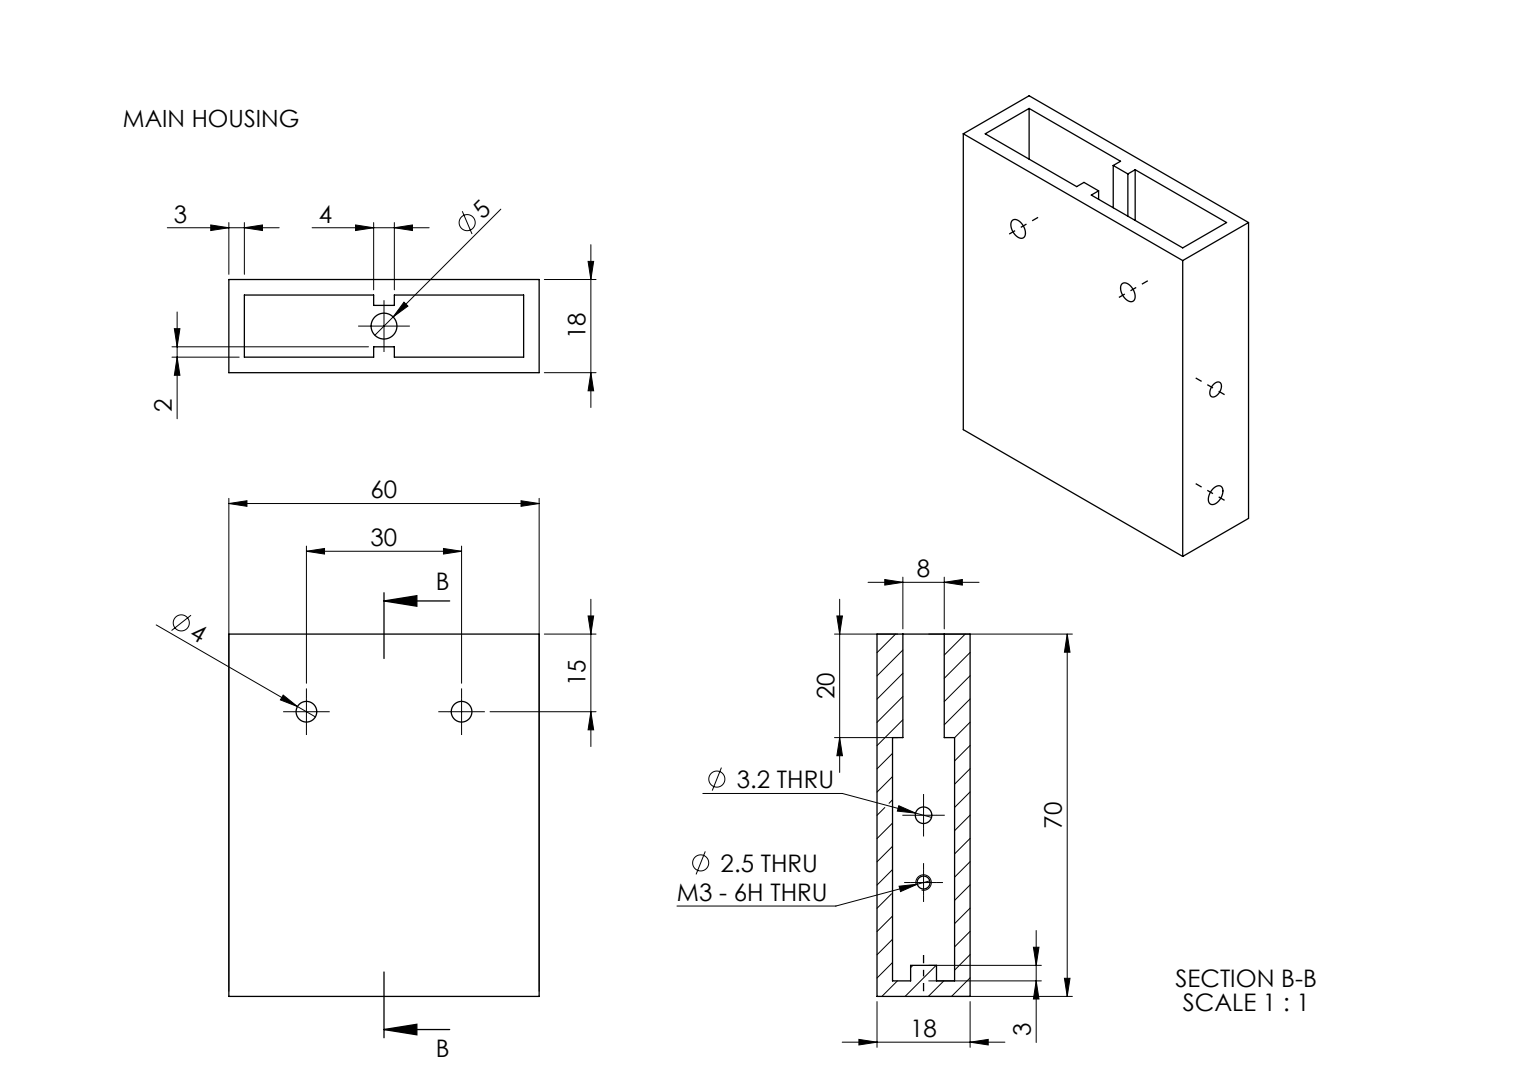
ISO-10303-21;
HEADER;
FILE_DESCRIPTION (('STEP AP214'),
    '1' );
FILE_NAME ('main housing.step',
    '2026-10-03T18:28:46',
    ( '' ),
    ( '' ),
    'SwSTEP 2.0',
    'SolidWorks 2026',
    '' );
FILE_SCHEMA (( 'AUTOMOTIVE_DESIGN' ));
ENDSEC;

DATA;
#38=CARTESIAN_POINT ( 'NONE',  ( 7.054542135639013677E-15, -28.99999999999999289, 0.000000000000000000 ) ) ;
#48=VERTEX_POINT ( 'NONE', #8977 ) ;
#68=DIRECTION ( 'NONE',  ( 0.000000000000000000, -0.000000000000000000, 1.000000000000000000 ) ) ;
#80=PRODUCT_DEFINITION_CONTEXT ( 'detailed design', #6135, 'design' ) ;
#82=PLANE ( 'NONE',  #8867 ) ;
#92=ORIENTED_EDGE ( 'NONE', *, *, #6887, .T. ) ;
#105=ORIENTED_EDGE ( 'NONE', *, *, #5645, .T. ) ;
#118=VERTEX_POINT ( 'NONE', #6579 ) ;
#125=CARTESIAN_POINT ( 'NONE',  ( 30.00000000000001066, -34.99999999999999289, -9.000000000000000000 ) ) ;
#137=DIRECTION ( 'NONE',  ( 5.204170427930421283E-15, 6.018531076210112041E-31, 1.000000000000000000 ) ) ;
#159=CARTESIAN_POINT ( 'NONE',  ( 1.999999999999987121, 15.00000000000000355, 4.000000000000008882 ) ) ;
#183=AXIS2_PLACEMENT_3D ( 'NONE', #2466, #1616, #8926 ) ;
#189=DIRECTION ( 'NONE',  ( 1.000000000000000000, 1.156482317317871478E-16, 5.637851296924623057E-15 ) ) ;
#199=VECTOR ( 'NONE', #189, 1000.000000000000000 ) ;
#205=DIRECTION ( 'NONE',  ( 0.000000000000000000, 0.000000000000000000, 1.000000000000000000 ) ) ;
#207=ORIENTED_EDGE ( 'NONE', *, *, #5389, .F. ) ;
#221=DIRECTION ( 'NONE',  ( -0.000000000000000000, -0.000000000000000000, 1.000000000000000000 ) ) ;
#225=CYLINDRICAL_SURFACE ( 'NONE', #1715, 2.500000000000000000 ) ;
#233=EDGE_CURVE ( 'NONE', #10188, #6283, #1978, .T. ) ;
#236=DIRECTION ( 'NONE',  ( -0.000000000000000000, -0.000000000000000000, 1.000000000000000000 ) ) ;
#269=ORIENTED_EDGE ( 'NONE', *, *, #2906, .F. ) ;
#278=PLANE ( 'NONE',  #8859 ) ;
#292=VERTEX_POINT ( 'NONE', #4247 ) ;
#294=DIRECTION ( 'NONE',  ( 0.000000000000000000, 0.000000000000000000, -1.000000000000000000 ) ) ;
#302=ORIENTED_EDGE ( 'NONE', *, *, #6506, .F. ) ;
#317=VERTEX_POINT ( 'NONE', #6837 ) ;
#322=ORIENTED_EDGE ( 'NONE', *, *, #3486, .F. ) ;
#331=DIRECTION ( 'NONE',  ( -1.000000000000000000, -4.625929269271485914E-16, 0.000000000000000000 ) ) ;
#341=VECTOR ( 'NONE', #1990, 1000.000000000000000 ) ;
#353=EDGE_CURVE ( 'NONE', #8450, #9806, #2322, .T. ) ;
#373=DIRECTION ( 'NONE',  ( 1.000000000000000000, -0.000000000000000000, -0.000000000000000000 ) ) ;
#386=CARTESIAN_POINT ( 'NONE',  ( 15.00000000000000000, 19.99999999999999645, -9.000000000000000000 ) ) ;
#397=AXIS2_PLACEMENT_3D ( 'NONE', #6365, #7050, #5039 ) ;
#398=EDGE_CURVE ( 'NONE', #7355, #525, #6229, .T. ) ;
#407=LINE ( 'NONE', #6055, #6780 ) ;
#409=VERTEX_POINT ( 'NONE', #6198 ) ;
#426=ORIENTED_EDGE ( 'NONE', *, *, #10066, .T. ) ;
#437=FACE_OUTER_BOUND ( 'NONE', #3682, .T. ) ;
#447=EDGE_CURVE ( 'NONE', #6622, #1459, #1384, .T. ) ;
#459=ORIENTED_EDGE ( 'NONE', *, *, #8953, .F. ) ;
#465=UNCERTAINTY_MEASURE_WITH_UNIT (LENGTH_MEASURE( 1.000000000000000082E-05 ), #9812, 'distance_accuracy_value', 'NONE');
#471=FACE_OUTER_BOUND ( 'NONE', #5653, .T. ) ;
#492=AXIS2_PLACEMENT_3D ( 'NONE', #2926, #2979, #637 ) ;
#512=ORIENTED_EDGE ( 'NONE', *, *, #4233, .T. ) ;
#516=AXIS2_PLACEMENT_3D ( 'NONE', #386, #236, #2717 ) ;
#522=VECTOR ( 'NONE', #7006, 1000.000000000000000 ) ;
#523=FACE_OUTER_BOUND ( 'NONE', #2494, .T. ) ;
#525=VERTEX_POINT ( 'NONE', #8496 ) ;
#530=ADVANCED_FACE ( 'NONE', ( #437 ), #3663, .F. ) ;
#533=SURFACE_SIDE_STYLE ('',( #7795 ) ) ;
#536=DIRECTION ( 'NONE',  ( 1.000000000000000000, 0.000000000000000000, 0.000000000000000000 ) ) ;
#541=EDGE_CURVE ( 'NONE', #3837, #9529, #1280, .T. ) ;
#556=ORIENTED_EDGE ( 'NONE', *, *, #8304, .F. ) ;
#565=EDGE_LOOP ( 'NONE', ( #3549, #2681, #8103, #9350 ) ) ;
#570=LINE ( 'NONE', #3276, #6753 ) ;
#576=CIRCLE ( 'NONE', #8201, 2.000000000000001776 ) ;
#585=CARTESIAN_POINT ( 'NONE',  ( 30.00000000000001066, -31.99999999999998579, 9.000000000000000000 ) ) ;
#597=LINE ( 'NONE', #648, #8239 ) ;
#617=DIRECTION ( 'NONE',  ( -0.000000000000000000, -0.000000000000000000, 1.000000000000000000 ) ) ;
#622=ORIENTED_EDGE ( 'NONE', *, *, #4233, .F. ) ;
#635=DIRECTION ( 'NONE',  ( -0.000000000000000000, -0.000000000000000000, 1.000000000000000000 ) ) ;
#636=FACE_BOUND ( 'NONE', #3921, .T. ) ;
#637=DIRECTION ( 'NONE',  ( 0.000000000000000000, 0.000000000000000000, 1.000000000000000000 ) ) ;
#648=CARTESIAN_POINT ( 'NONE',  ( 1.999999999999986233, 15.00000000000000355, -4.000000000000009770 ) ) ;
#659=ORIENTED_EDGE ( 'NONE', *, *, #7728, .T. ) ;
#662=ORIENTED_EDGE ( 'NONE', *, *, #2847, .T. ) ;
#668=AXIS2_PLACEMENT_3D ( 'NONE', #5379, #617, #3899 ) ;
#676=LINE ( 'NONE', #2269, #8398 ) ;
#681=DIRECTION ( 'NONE',  ( -1.156482317317871478E-16, 1.000000000000000000, 0.000000000000000000 ) ) ;
#688=SURFACE_STYLE_USAGE ( .BOTH. , #533 ) ;
#692=CARTESIAN_POINT ( 'NONE',  ( -2.000000000000015099, 35.00000000000000000, 3.999999999999986233 ) ) ;
#696=DIRECTION ( 'NONE',  ( -1.000000000000000000, -2.312964634635742957E-16, 0.000000000000000000 ) ) ;
#701=VECTOR ( 'NONE', #1350, 1000.000000000000000 ) ;
#713=DIRECTION ( 'NONE',  ( 1.156482317317871478E-16, -1.000000000000000000, 0.000000000000000000 ) ) ;
#714=CARTESIAN_POINT ( 'NONE',  ( -13.00000000000000000, 19.99999999999999645, -9.000000000000000000 ) ) ;
#724=ORIENTED_EDGE ( 'NONE', *, *, #8186, .F. ) ;
#730=AXIS2_PLACEMENT_3D ( 'NONE', #6023, #9492, #6879 ) ;
#746=FACE_OUTER_BOUND ( 'NONE', #9469, .T. ) ;
#761=DIRECTION ( 'NONE',  ( 4.625929269271485914E-16, -1.000000000000000000, 0.000000000000000000 ) ) ;
#762=CARTESIAN_POINT ( 'NONE',  ( 30.00000000000001066, 35.00000000000001421, 5.999999999999999112 ) ) ;
#772=ORIENTED_EDGE ( 'NONE', *, *, #3509, .F. ) ;
#778=CARTESIAN_POINT ( 'NONE',  ( -29.99999999999998934, -35.00000000000000000, 9.000000000000000000 ) ) ;
#781=VECTOR ( 'NONE', #5041, 1000.000000000000000 ) ;
#805=EDGE_LOOP ( 'NONE', ( #3050, #7525, #1781, #3634 ) ) ;
#834=LINE ( 'NONE', #4066, #3644 ) ;
#867=CIRCLE ( 'NONE', #2217, 1.999999999999997780 ) ;
#870=CYLINDRICAL_SURFACE ( 'NONE', #6948, 1.599999999999998979 ) ;
#875=CARTESIAN_POINT ( 'NONE',  ( -2.499999999999992895, -31.99999999999999289, 3.061616997868383141E-16 ) ) ;
#880=ORIENTED_EDGE ( 'NONE', *, *, #4483, .T. ) ;
#887=FACE_OUTER_BOUND ( 'NONE', #7832, .T. ) ;
#900=ORIENTED_EDGE ( 'NONE', *, *, #447, .F. ) ;
#916=DIRECTION ( 'NONE',  ( 0.000000000000000000, 0.000000000000000000, 1.000000000000000000 ) ) ;
#921=AXIS2_PLACEMENT_3D ( 'NONE', #4394, #3705, #6721 ) ;
#923=CARTESIAN_POINT ( 'NONE',  ( 30.00000000000001066, -34.99999999999999289, 9.000000000000000000 ) ) ;
#953=VECTOR ( 'NONE', #9625, 1000.000000000000000 ) ;
#970=CARTESIAN_POINT ( 'NONE',  ( 30.00000000000001066, 35.00000000000001421, 5.999999999999999112 ) ) ;
#973=ADVANCED_FACE ( 'NONE', ( #4956, #8202, #3210 ), #1831, .F. ) ;
#975=CARTESIAN_POINT ( 'NONE',  ( 30.00000000000001066, -31.99999999999998579, -6.000000000000000000 ) ) ;
#990=CARTESIAN_POINT ( 'NONE',  ( -29.99999999999998934, -13.00000000000000533, 1.249999999999993339 ) ) ;
#1009=CARTESIAN_POINT ( 'NONE',  ( -29.99999999999998934, 0.000000000000000000, 0.000000000000000000 ) ) ;
#1014=CIRCLE ( 'NONE', #9484, 2.500000000000000000 ) ;
#1035=ORIENTED_EDGE ( 'NONE', *, *, #7193, .T. ) ;
#1039=EDGE_LOOP ( 'NONE', ( #4958, #5026 ) ) ;
#1041=AXIS2_PLACEMENT_3D ( 'NONE', #6956, #8405, #294 ) ;
#1046=DIRECTION ( 'NONE',  ( -0.000000000000000000, -0.000000000000000000, -1.000000000000000000 ) ) ;
#1069=EDGE_CURVE ( 'NONE', #3641, #9420, #7060, .T. ) ;
#1085=AXIS2_PLACEMENT_3D ( 'NONE', #9340, #1919, #1275 ) ;
#1103=ADVANCED_FACE ( 'NONE', ( #7979 ), #5367, .T. ) ;
#1108=ORIENTED_EDGE ( 'NONE', *, *, #9516, .F. ) ;
#1114=EDGE_LOOP ( 'NONE', ( #5375, #5317, #9863, #4627 ) ) ;
#1132=ORIENTED_EDGE ( 'NONE', *, *, #3008, .T. ) ;
#1141=ORIENTED_EDGE ( 'NONE', *, *, #1425, .T. ) ;
#1150=ORIENTED_EDGE ( 'NONE', *, *, #5004, .T. ) ;
#1166=FACE_BOUND ( 'NONE', #3116, .T. ) ;
#1185=DIRECTION ( 'NONE',  ( 0.000000000000000000, 0.000000000000000000, -1.000000000000000000 ) ) ;
#1189=CARTESIAN_POINT ( 'NONE',  ( -29.99999999999998934, -35.00000000000000000, -9.000000000000000000 ) ) ;
#1196=ORIENTED_EDGE ( 'NONE', *, *, #1425, .F. ) ;
#1197=EDGE_CURVE ( 'NONE', #8501, #9821, #4045, .T. ) ;
#1201=DIRECTION ( 'NONE',  ( 1.000000000000000000, 0.000000000000000000, 0.000000000000000000 ) ) ;
#1211=VERTEX_POINT ( 'NONE', #875 ) ;
#1220=LINE ( 'NONE', #4499, #6090 ) ;
#1222=FACE_BOUND ( 'NONE', #1039, .T. ) ;
#1225=CYLINDRICAL_SURFACE ( 'NONE', #2645, 2.000000000000000000 ) ;
#1242=CIRCLE ( 'NONE', #1595, 2.000000000000001776 ) ;
#1243=DIRECTION ( 'NONE',  ( -0.000000000000000000, -0.000000000000000000, 1.000000000000000000 ) ) ;
#1250=DIRECTION ( 'NONE',  ( -0.000000000000000000, -1.000000000000000000, -0.000000000000000000 ) ) ;
#1251=DIRECTION ( 'NONE',  ( -1.000000000000000000, -1.156482317317871478E-16, 5.204170427930421283E-15 ) ) ;
#1252=DIRECTION ( 'NONE',  ( 0.000000000000000000, -0.000000000000000000, 1.000000000000000000 ) ) ;
#1253=ORIENTED_EDGE ( 'NONE', *, *, #7964, .T. ) ;
#1257=ORIENTED_EDGE ( 'NONE', *, *, #398, .T. ) ;
#1262=CARTESIAN_POINT ( 'NONE',  ( 27.00000000000001066, -25.00000000000000000, 1.999999999999997780 ) ) ;
#1275=DIRECTION ( 'NONE',  ( 0.000000000000000000, 0.000000000000000000, 1.000000000000000000 ) ) ;
#1280=LINE ( 'NONE', #4506, #5723 ) ;
#1285=AXIS2_PLACEMENT_3D ( 'NONE', #7974, #761, #8821 ) ;
#1297=ORIENTED_EDGE ( 'NONE', *, *, #1971, .T. ) ;
#1298=ORIENTED_EDGE ( 'NONE', *, *, #1579, .T. ) ;
#1302=ADVANCED_FACE ( 'NONE', ( #9188 ), #9943, .F. ) ;
#1306=ORIENTED_EDGE ( 'NONE', *, *, #3124, .F. ) ;
#1311=CARTESIAN_POINT ( 'NONE',  ( 15.00000000000000000, 19.99999999999999645, -5.999999999999999112 ) ) ;
#1313=ORIENTED_EDGE ( 'NONE', *, *, #8953, .T. ) ;
#1314=ADVANCED_FACE ( 'NONE', ( #1926 ), #8447, .F. ) ;
#1335=MECHANICAL_DESIGN_GEOMETRIC_PRESENTATION_REPRESENTATION('',(#7777),#1870);
#1337=FACE_OUTER_BOUND ( 'NONE', #8575, .T. ) ;
#1338=ORIENTED_EDGE ( 'NONE', *, *, #6493, .T. ) ;
#1350=DIRECTION ( 'NONE',  ( 0.000000000000000000, 0.000000000000000000, -1.000000000000000000 ) ) ;
#1360=VECTOR ( 'NONE', #3934, 1000.000000000000000 ) ;
#1367=ORIENTED_EDGE ( 'NONE', *, *, #7316, .T. ) ;
#1373=DIRECTION ( 'NONE',  ( 1.000000000000000000, -0.000000000000000000, -0.000000000000000000 ) ) ;
#1375=DIRECTION ( 'NONE',  ( 0.000000000000000000, 0.000000000000000000, 1.000000000000000000 ) ) ;
#1377=EDGE_CURVE ( 'NONE', #9102, #6283, #3929, .T. ) ;
#1384=LINE ( 'NONE', #10246, #4886 ) ;
#1389=PLANE ( 'NONE',  #397 ) ;
#1395=LINE ( 'NONE', #762, #4577 ) ;
#1398=LINE ( 'NONE', #6160, #5914 ) ;
#1409=DIRECTION ( 'NONE',  ( -1.156482317317871478E-16, 1.000000000000000000, 0.000000000000000000 ) ) ;
#1413=EDGE_LOOP ( 'NONE', ( #3627, #3535, #1150, #6040 ) ) ;
#1418=LINE ( 'NONE', #4644, #3557 ) ;
#1423=ORIENTED_EDGE ( 'NONE', *, *, #6274, .F. ) ;
#1425=EDGE_CURVE ( 'NONE', #9585, #6050, #867, .T. ) ;
#1432=DIRECTION ( 'NONE',  ( 5.204170427930421283E-15, 0.000000000000000000, 1.000000000000000000 ) ) ;
#1440=DIRECTION ( 'NONE',  ( 0.000000000000000000, 0.000000000000000000, -1.000000000000000000 ) ) ;
#1459=VERTEX_POINT ( 'NONE', #9878 ) ;
#1474=ORIENTED_EDGE ( 'NONE', *, *, #7964, .F. ) ;
#1480=ADVANCED_FACE ( 'NONE', ( #7485 ), #5244, .F. ) ;
#1502=ORIENTED_EDGE ( 'NONE', *, *, #4674, .F. ) ;
#1505=EDGE_LOOP ( 'NONE', ( #2316, #3449, #2852, #4065 ) ) ;
#1524=DIRECTION ( 'NONE',  ( -1.000000000000000000, 0.000000000000000000, 0.000000000000000000 ) ) ;
#1555=ADVANCED_FACE ( 'NONE', ( #3551 ), #225, .T. ) ;
#1566=CARTESIAN_POINT ( 'NONE',  ( 12.99999999999999645, 19.99999999999999645, -5.999999999999999112 ) ) ;
#1572=ORIENTED_EDGE ( 'NONE', *, *, #8813, .F. ) ;
#1577=FACE_BOUND ( 'NONE', #5153, .T. ) ;
#1579=EDGE_CURVE ( 'NONE', #8329, #6538, #9123, .T. ) ;
#1590=LINE ( 'NONE', #9652, #7504 ) ;
#1595=AXIS2_PLACEMENT_3D ( 'NONE', #5090, #2660, #3294 ) ;
#1596=( NAMED_UNIT ( * ) PLANE_ANGLE_UNIT ( ) SI_UNIT ( $, .RADIAN. ) );
#1599=LINE ( 'NONE', #4873, #8156 ) ;
#1601=CARTESIAN_POINT ( 'NONE',  ( -26.99999999999998934, -32.00000000000000000, -5.999999999999999112 ) ) ;
#1612=CARTESIAN_POINT ( 'NONE',  ( 7.401486830834375884E-15, -31.99999999999999289, 0.000000000000000000 ) ) ;
#1616=DIRECTION ( 'NONE',  ( -1.000000000000000000, -1.156482317317871478E-16, -5.694029147589358720E-15 ) ) ;
#1623=AXIS2_PLACEMENT_3D ( 'NONE', #1311, #3909, #3796 ) ;
#1638=CARTESIAN_POINT ( 'NONE',  ( 27.00000000000001066, -34.99999999999999289, 5.999999999999999112 ) ) ;
#1656=LINE ( 'NONE', #9933, #5135 ) ;
#1701=CARTESIAN_POINT ( 'NONE',  ( 30.00000000000001066, 0.000000000000000000, 0.000000000000000000 ) ) ;
#1702=CIRCLE ( 'NONE', #6762, 2.000000000000000000 ) ;
#1708=EDGE_CURVE ( 'NONE', #3161, #7840, #1220, .T. ) ;
#1715=AXIS2_PLACEMENT_3D ( 'NONE', #10086, #6776, #2813 ) ;
#1717=FACE_BOUND ( 'NONE', #2962, .T. ) ;
#1733=ORIENTED_EDGE ( 'NONE', *, *, #2258, .T. ) ;
#1747=VERTEX_POINT ( 'NONE', #3806 ) ;
#1772=CARTESIAN_POINT ( 'NONE',  ( 15.00000000000000000, 19.99999999999999645, -9.000000000000000000 ) ) ;
#1781=ORIENTED_EDGE ( 'NONE', *, *, #6468, .T. ) ;
#1782=CIRCLE ( 'NONE', #7705, 1.599999999999992983 ) ;
#1790=CIRCLE ( 'NONE', #3138, 1.599999999999992983 ) ;
#1793=DIRECTION ( 'NONE',  ( -1.000000000000000000, -1.156482317317871478E-16, 0.000000000000000000 ) ) ;
#1803=DIRECTION ( 'NONE',  ( -5.694029147589358720E-15, -6.585044023479645679E-31, 1.000000000000000000 ) ) ;
#1828=DIRECTION ( 'NONE',  ( -1.000000000000000000, -0.000000000000000000, -0.000000000000000000 ) ) ;
#1829=DIRECTION ( 'NONE',  ( -1.000000000000000000, 0.000000000000000000, 0.000000000000000000 ) ) ;
#1831=PLANE ( 'NONE',  #5231 ) ;
#1833=ORIENTED_EDGE ( 'NONE', *, *, #6506, .T. ) ;
#1855=AXIS2_PLACEMENT_3D ( 'NONE', #8574, #7021, #4689 ) ;
#1863=CARTESIAN_POINT ( 'NONE',  ( -17.00000000000000000, 19.99999999999999645, -9.000000000000000000 ) ) ;
#1870=( GEOMETRIC_REPRESENTATION_CONTEXT ( 3 ) GLOBAL_UNCERTAINTY_ASSIGNED_CONTEXT ( ( #3256 ) ) GLOBAL_UNIT_ASSIGNED_CONTEXT ( ( #8779, #8724, #8618 ) ) REPRESENTATION_CONTEXT ( 'NONE', 'WORKASPACE' ) );
#1875=CIRCLE ( 'NONE', #9672, 1.599999999999998979 ) ;
#1877=FACE_BOUND ( 'NONE', #7579, .T. ) ;
#1881=AXIS2_PLACEMENT_3D ( 'NONE', #8069, #8855, #3978 ) ;
#1890=VECTOR ( 'NONE', #1828, 1000.000000000000000 ) ;
#1891=DIRECTION ( 'NONE',  ( 1.000000000000000000, 0.000000000000000000, 0.000000000000000000 ) ) ;
#1919=DIRECTION ( 'NONE',  ( -1.000000000000000000, -0.000000000000000000, -0.000000000000000000 ) ) ;
#1926=FACE_OUTER_BOUND ( 'NONE', #3493, .T. ) ;
#1934=CARTESIAN_POINT ( 'NONE',  ( -26.99999999999998934, 34.99999999999999289, 5.999999999999999112 ) ) ;
#1936=CIRCLE ( 'NONE', #3614, 2.000000000000000000 ) ;
#1947=DIRECTION ( 'NONE',  ( 0.000000000000000000, 0.000000000000000000, -1.000000000000000000 ) ) ;
#1948=ORIENTED_EDGE ( 'NONE', *, *, #6566, .T. ) ;
#1955=VECTOR ( 'NONE', #4995, 1000.000000000000000 ) ;
#1963=VECTOR ( 'NONE', #2407, 1000.000000000000000 ) ;
#1964=DIRECTION ( 'NONE',  ( -1.000000000000000000, 0.000000000000000000, 0.000000000000000000 ) ) ;
#1971=EDGE_CURVE ( 'NONE', #5116, #1459, #3575, .T. ) ;
#1973=CIRCLE ( 'NONE', #6013, 2.000000000000000000 ) ;
#1978=LINE ( 'NONE', #970, #3384 ) ;
#1990=DIRECTION ( 'NONE',  ( -0.000000000000000000, -1.000000000000000000, -0.000000000000000000 ) ) ;
#1999=CARTESIAN_POINT ( 'NONE',  ( -2.499999999999992895, -28.99999999999999289, 3.061616997868383141E-16 ) ) ;
#2001=VERTEX_POINT ( 'NONE', #5594 ) ;
#2011=ORIENTED_EDGE ( 'NONE', *, *, #8140, .T. ) ;
#2020=DIRECTION ( 'NONE',  ( 0.000000000000000000, 0.000000000000000000, 1.000000000000000000 ) ) ;
#2022=CARTESIAN_POINT ( 'NONE',  ( -15.00000000000000000, 19.99999999999999645, -9.000000000000000000 ) ) ;
#2034=VERTEX_POINT ( 'NONE', #3109 ) ;
#2049=EDGE_LOOP ( 'NONE', ( #4459, #1298, #8039, #4474 ) ) ;
#2053=DIRECTION ( 'NONE',  ( 0.000000000000000000, -0.000000000000000000, 1.000000000000000000 ) ) ;
#2066=ORIENTED_EDGE ( 'NONE', *, *, #10380, .T. ) ;
#2079=DIRECTION ( 'NONE',  ( -1.000000000000000000, -0.000000000000000000, -0.000000000000000000 ) ) ;
#2101=AXIS2_PLACEMENT_3D ( 'NONE', #7090, #5610, #4547 ) ;
#2113=PLANE ( 'NONE',  #6176 ) ;
#2130=CARTESIAN_POINT ( 'NONE',  ( -2.000000000000015099, 35.00000000000000000, 3.999999999999986233 ) ) ;
#2135=VECTOR ( 'NONE', #1250, 1000.000000000000000 ) ;
#2144=CARTESIAN_POINT ( 'NONE',  ( 17.00000000000000000, 19.99999999999999645, -5.999999999999999112 ) ) ;
#2157=SURFACE_SIDE_STYLE ('',( #5485 ) ) ;
#2164=DIRECTION ( 'NONE',  ( 0.000000000000000000, 0.000000000000000000, 1.000000000000000000 ) ) ;
#2209=CARTESIAN_POINT ( 'NONE',  ( -2.000000000000012879, 15.00000000000000355, 3.999999999999986233 ) ) ;
#2210=VERTEX_POINT ( 'NONE', #3829 ) ;
#2217=AXIS2_PLACEMENT_3D ( 'NONE', #4985, #2341, #4776 ) ;
#2219=CARTESIAN_POINT ( 'NONE',  ( 27.00000000000001066, 0.000000000000000000, 0.000000000000000000 ) ) ;
#2232=EDGE_CURVE ( 'NONE', #8002, #7355, #7917, .T. ) ;
#2237=DIRECTION ( 'NONE',  ( -0.000000000000000000, -0.000000000000000000, 1.000000000000000000 ) ) ;
#2257=CIRCLE ( 'NONE', #8024, 2.000000000000000000 ) ;
#2258=EDGE_CURVE ( 'NONE', #9806, #9585, #1599, .T. ) ;
#2269=CARTESIAN_POINT ( 'NONE',  ( -29.99999999999998934, 34.99999999999999289, 9.000000000000000000 ) ) ;
#2270=CARTESIAN_POINT ( 'NONE',  ( 30.00000000000001066, 1.959434878635752904E-16, 1.599999999999986766 ) ) ;
#2280=LINE ( 'NONE', #3973, #9051 ) ;
#2281=ORIENTED_EDGE ( 'NONE', *, *, #7853, .F. ) ;
#2284=CARTESIAN_POINT ( 'NONE',  ( -29.99999999999998934, 1.959434878635763751E-16, -1.599999999999998979 ) ) ;
#2300=CARTESIAN_POINT ( 'NONE',  ( 27.00000000000001066, 1.959434878635756602E-16, 1.599999999999992983 ) ) ;
#2316=ORIENTED_EDGE ( 'NONE', *, *, #2232, .F. ) ;
#2319=EDGE_LOOP ( 'NONE', ( #7682, #7519, #8207, #1253 ) ) ;
#2320=EDGE_LOOP ( 'NONE', ( #3515, #662, #3143, #3332 ) ) ;
#2321=CARTESIAN_POINT ( 'NONE',  ( 30.00000000000001066, -31.99999999999998579, 5.999999999999999112 ) ) ;
#2322=CIRCLE ( 'NONE', #3922, 1.999999999999997780 ) ;
#2331=DIRECTION ( 'NONE',  ( 1.000000000000000000, 0.000000000000000000, 0.000000000000000000 ) ) ;
#2335=CARTESIAN_POINT ( 'NONE',  ( -2.000000000000024425, 15.00000000000000355, 5.999999999999987566 ) ) ;
#2336=CARTESIAN_POINT ( 'NONE',  ( -15.00000000000000000, 19.99999999999999645, -9.000000000000000000 ) ) ;
#2341=DIRECTION ( 'NONE',  ( 1.000000000000000000, 0.000000000000000000, 0.000000000000000000 ) ) ;
#2348=ADVANCED_FACE ( 'NONE', ( #7317 ), #8908, .F. ) ;
#2362=EDGE_CURVE ( 'NONE', #7675, #9850, #7807, .T. ) ;
#2384=VECTOR ( 'NONE', #9630, 1000.000000000000000 ) ;
#2386=( LENGTH_UNIT ( ) NAMED_UNIT ( * ) SI_UNIT ( .MILLI., .METRE. ) );
#2387=ORIENTED_EDGE ( 'NONE', *, *, #4483, .F. ) ;
#2393=FACE_OUTER_BOUND ( 'NONE', #8936, .T. ) ;
#2400=CIRCLE ( 'NONE', #1041, 1.599999999999986766 ) ;
#2404=EDGE_LOOP ( 'NONE', ( #2281, #9067 ) ) ;
#2407=DIRECTION ( 'NONE',  ( -1.156482317317871478E-16, 1.000000000000000000, 0.000000000000000000 ) ) ;
#2422=CARTESIAN_POINT ( 'NONE',  ( 7.054542135639013677E-15, -28.99999999999999289, 0.000000000000000000 ) ) ;
#2441=CIRCLE ( 'NONE', #9892, 2.000000000000003553 ) ;
#2442=ADVANCED_FACE ( 'NONE', ( #2949 ), #5218, .F. ) ;
#2444=VERTEX_POINT ( 'NONE', #7478 ) ;
#2457=EDGE_CURVE ( 'NONE', #2653, #1211, #2839, .T. ) ;
#2462=DIRECTION ( 'NONE',  ( 0.000000000000000000, 0.000000000000000000, 1.000000000000000000 ) ) ;
#2466=CARTESIAN_POINT ( 'NONE',  ( -2.000000000000012879, 15.00000000000000355, 3.999999999999986233 ) ) ;
#2488=EDGE_CURVE ( 'NONE', #9102, #5109, #407, .T. ) ;
#2494=EDGE_LOOP ( 'NONE', ( #8137, #10442, #1297, #900 ) ) ;
#2497=DIRECTION ( 'NONE',  ( 1.000000000000000000, 0.000000000000000000, 0.000000000000000000 ) ) ;
#2499=FACE_OUTER_BOUND ( 'NONE', #1114, .T. ) ;
#2502=ORIENTED_EDGE ( 'NONE', *, *, #6178, .T. ) ;
#2505=CARTESIAN_POINT ( 'NONE',  ( 15.00000000000000000, 19.99999999999999645, 6.000000000000000000 ) ) ;
#2521=ORIENTED_EDGE ( 'NONE', *, *, #6093, .F. ) ;
#2524=ORIENTED_EDGE ( 'NONE', *, *, #9868, .T. ) ;
#2528=VERTEX_POINT ( 'NONE', #3001 ) ;
#2532=LINE ( 'NONE', #5020, #5671 ) ;
#2533=AXIS2_PLACEMENT_3D ( 'NONE', #9412, #713, #3148 ) ;
#2542=VECTOR ( 'NONE', #10396, 1000.000000000000000 ) ;
#2543=EDGE_CURVE ( 'NONE', #8501, #292, #5326, .T. ) ;
#2548=PLANE ( 'NONE',  #5074 ) ;
#2555=DIRECTION ( 'NONE',  ( -1.156482317317871478E-16, 1.000000000000000000, 0.000000000000000000 ) ) ;
#2578=CARTESIAN_POINT ( 'NONE',  ( 0.000000000000000000, 0.000000000000000000, 5.999999999999999112 ) ) ;
#2579=VERTEX_POINT ( 'NONE', #7015 ) ;
#2635=AXIS2_PLACEMENT_3D ( 'NONE', #6766, #10075, #2164 ) ;
#2645=AXIS2_PLACEMENT_3D ( 'NONE', #4504, #3814, #2819 ) ;
#2647=VECTOR ( 'NONE', #3350, 1000.000000000000000 ) ;
#2650=EDGE_CURVE ( 'NONE', #5636, #525, #5431, .T. ) ;
#2652=DIRECTION ( 'NONE',  ( -5.694029147589358720E-15, -6.585044023479645679E-31, 1.000000000000000000 ) ) ;
#2653=VERTEX_POINT ( 'NONE', #4740 ) ;
#2654=CARTESIAN_POINT ( 'NONE',  ( 30.00000000000001066, 0.000000000000000000, 0.000000000000000000 ) ) ;
#2660=DIRECTION ( 'NONE',  ( 0.000000000000000000, -0.000000000000000000, 1.000000000000000000 ) ) ;
#2662=EDGE_CURVE ( 'NONE', #10188, #2753, #3156, .T. ) ;
#2663=CARTESIAN_POINT ( 'NONE',  ( -26.99999999999998579, -32.00000000000000000, 9.000000000000000000 ) ) ;
#2681=ORIENTED_EDGE ( 'NONE', *, *, #9656, .F. ) ;
#2685=DIRECTION ( 'NONE',  ( 1.000000000000000000, -0.000000000000000000, -0.000000000000000000 ) ) ;
#2697=CARTESIAN_POINT ( 'NONE',  ( 15.00000000000000000, 19.99999999999999645, -9.000000000000000000 ) ) ;
#2717=DIRECTION ( 'NONE',  ( 1.000000000000000000, 0.000000000000000000, 0.000000000000000000 ) ) ;
#2722=AXIS2_PLACEMENT_3D ( 'NONE', #3461, #5099, #7702 ) ;
#2725=VECTOR ( 'NONE', #4629, 1000.000000000000000 ) ;
#2740=ORIENTED_EDGE ( 'NONE', *, *, #3234, .F. ) ;
#2753=VERTEX_POINT ( 'NONE', #3103 ) ;
#2766=CARTESIAN_POINT ( 'NONE',  ( 27.00000000000001066, -25.00000000000000000, 0.000000000000000000 ) ) ;
#2778=DIRECTION ( 'NONE',  ( 1.000000000000000000, 0.000000000000000000, 0.000000000000000000 ) ) ;
#2779=ORIENTED_EDGE ( 'NONE', *, *, #6684, .F. ) ;
#2798=CIRCLE ( 'NONE', #1623, 2.000000000000001776 ) ;
#2803=EDGE_CURVE ( 'NONE', #3690, #48, #6692, .T. ) ;
#2804=DIRECTION ( 'NONE',  ( -5.637851296924623057E-15, -6.520075332560955295E-31, 1.000000000000000000 ) ) ;
#2806=FACE_OUTER_BOUND ( 'NONE', #2320, .T. ) ;
#2811=ORIENTED_EDGE ( 'NONE', *, *, #9703, .F. ) ;
#2813=DIRECTION ( 'NONE',  ( 1.000000000000000000, 0.000000000000000000, 0.000000000000000000 ) ) ;
#2819=DIRECTION ( 'NONE',  ( 1.000000000000000000, 0.000000000000000000, 0.000000000000000000 ) ) ;
#2839=LINE ( 'NONE', #1999, #5763 ) ;
#2840=CARTESIAN_POINT ( 'NONE',  ( -15.00000000000000000, 19.99999999999999645, 6.000000000000000000 ) ) ;
#2847=EDGE_CURVE ( 'NONE', #9902, #7878, #4204, .T. ) ;
#2852=ORIENTED_EDGE ( 'NONE', *, *, #2650, .T. ) ;
#2879=LINE ( 'NONE', #9194, #5845 ) ;
#2883=DIRECTION ( 'NONE',  ( -0.000000000000000000, -0.000000000000000000, 1.000000000000000000 ) ) ;
#2891=VERTEX_POINT ( 'NONE', #9896 ) ;
#2892=DIRECTION ( 'NONE',  ( 5.204170427930421283E-15, 6.018531076210112041E-31, 1.000000000000000000 ) ) ;
#2896=ORIENTED_EDGE ( 'NONE', *, *, #2906, .T. ) ;
#2906=EDGE_CURVE ( 'NONE', #2891, #5519, #4952, .T. ) ;
#2909=FACE_OUTER_BOUND ( 'NONE', #9860, .T. ) ;
#2926=CARTESIAN_POINT ( 'NONE',  ( -29.99999999999998934, 0.000000000000000000, 0.000000000000000000 ) ) ;
#2939=VERTEX_POINT ( 'NONE', #4514 ) ;
#2948=EDGE_CURVE ( 'NONE', #7840, #3946, #2400, .T. ) ;
#2949=FACE_OUTER_BOUND ( 'NONE', #8605, .T. ) ;
#2950=CARTESIAN_POINT ( 'NONE',  ( 1.999999999999987121, 15.00000000000000355, 4.000000000000008882 ) ) ;
#2961=CARTESIAN_POINT ( 'NONE',  ( -13.00000000000000000, 19.99999999999999645, 6.000000000000000000 ) ) ;
#2962=EDGE_LOOP ( 'NONE', ( #7083, #7502 ) ) ;
#2965=CARTESIAN_POINT ( 'NONE',  ( 17.00000000000000000, 19.99999999999999645, -9.000000000000000000 ) ) ;
#2979=DIRECTION ( 'NONE',  ( -1.000000000000000000, -0.000000000000000000, -0.000000000000000000 ) ) ;
#2990=FACE_BOUND ( 'NONE', #6798, .T. ) ;
#3001=CARTESIAN_POINT ( 'NONE',  ( -13.00000000000000000, 19.99999999999999645, -9.000000000000000000 ) ) ;
#3002=CARTESIAN_POINT ( 'NONE',  ( -29.99999999999998934, 34.99999999999999289, -9.000000000000000000 ) ) ;
#3008=EDGE_CURVE ( 'NONE', #2653, #3837, #10448, .T. ) ;
#3011=EDGE_LOOP ( 'NONE', ( #7772, #7066, #1257, #3387 ) ) ;
#3020=LINE ( 'NONE', #10347, #7178 ) ;
#3031=LINE ( 'NONE', #4038, #3771 ) ;
#3039=DIRECTION ( 'NONE',  ( -1.156482317317871478E-16, 1.000000000000000000, 0.000000000000000000 ) ) ;
#3043=EDGE_CURVE ( 'NONE', #5372, #292, #2879, .T. ) ;
#3044=DIRECTION ( 'NONE',  ( 5.204170427930421283E-15, 6.018531076210112041E-31, 1.000000000000000000 ) ) ;
#3050=ORIENTED_EDGE ( 'NONE', *, *, #5944, .F. ) ;
#3058=PRESENTATION_STYLE_ASSIGNMENT (( #7775 ) ) ;
#3065=LINE ( 'NONE', #1638, #2542 ) ;
#3078=CARTESIAN_POINT ( 'NONE',  ( 30.00000000000001066, 35.00000000000001421, -6.000000000000000000 ) ) ;
#3087=PRODUCT_CONTEXT ( 'NONE', #9064, 'mechanical' ) ;
#3090=EDGE_LOOP ( 'NONE', ( #512, #1108, #3371, #1338 ) ) ;
#3103=CARTESIAN_POINT ( 'NONE',  ( 27.00000000000001066, 35.00000000000001421, -5.999999999999999112 ) ) ;
#3109=CARTESIAN_POINT ( 'NONE',  ( -29.99999999999998934, 34.99999999999999289, 9.000000000000000000 ) ) ;
#3113=ORIENTED_EDGE ( 'NONE', *, *, #7728, .F. ) ;
#3114=DIRECTION ( 'NONE',  ( 0.000000000000000000, 0.000000000000000000, 1.000000000000000000 ) ) ;
#3116=EDGE_LOOP ( 'NONE', ( #2779, #5943 ) ) ;
#3117=CARTESIAN_POINT ( 'NONE',  ( 30.00000000000001066, -34.99999999999999289, -9.000000000000000000 ) ) ;
#3123=DIRECTION ( 'NONE',  ( -0.000000000000000000, -0.000000000000000000, -1.000000000000000000 ) ) ;
#3124=EDGE_CURVE ( 'NONE', #4718, #5808, #9764, .T. ) ;
#3138=AXIS2_PLACEMENT_3D ( 'NONE', #2219, #4807, #3114 ) ;
#3141=CARTESIAN_POINT ( 'NONE',  ( -2.000000000000019096, 35.00000000000000000, -6.000000000000000000 ) ) ;
#3143=ORIENTED_EDGE ( 'NONE', *, *, #10256, .T. ) ;
#3148=DIRECTION ( 'NONE',  ( -1.000000000000000000, -1.156482317317871478E-16, -0.000000000000000000 ) ) ;
#3154=ORIENTED_EDGE ( 'NONE', *, *, #9656, .T. ) ;
#3156=LINE ( 'NONE', #4848, #2725 ) ;
#3161=VERTEX_POINT ( 'NONE', #2300 ) ;
#3162=DIRECTION ( 'NONE',  ( 0.000000000000000000, 0.000000000000000000, 1.000000000000000000 ) ) ;
#3173=ORIENTED_EDGE ( 'NONE', *, *, #9523, .F. ) ;
#3177=( NAMED_UNIT ( * ) PLANE_ANGLE_UNIT ( ) SI_UNIT ( $, .RADIAN. ) );
#3179=PRODUCT_DEFINITION_SHAPE ( 'NONE', 'NONE',  #3345 ) ;
#3199=EDGE_CURVE ( 'NONE', #3641, #2001, #9519, .T. ) ;
#3205=ORIENTED_EDGE ( 'NONE', *, *, #3199, .T. ) ;
#3210=FACE_BOUND ( 'NONE', #7559, .T. ) ;
#3225=VECTOR ( 'NONE', #6435, 1000.000000000000000 ) ;
#3234=EDGE_CURVE ( 'NONE', #1747, #2210, #597, .T. ) ;
#3237=CARTESIAN_POINT ( 'NONE',  ( -17.00000000000000000, 19.99999999999999645, -9.000000000000000000 ) ) ;
#3248=ADVANCED_FACE ( 'NONE', ( #5573, #2990 ), #10307, .F. ) ;
#3256=UNCERTAINTY_MEASURE_WITH_UNIT (LENGTH_MEASURE( 1.000000000000000082E-05 ), #8779, 'distance_accuracy_value', 'NONE');
#3271=ORIENTED_EDGE ( 'NONE', *, *, #4674, .T. ) ;
#3276=CARTESIAN_POINT ( 'NONE',  ( -2.000000000000024425, 15.00000000000000355, 5.999999999999987566 ) ) ;
#3277=VERTEX_POINT ( 'NONE', #3938 ) ;
#3281=VERTEX_POINT ( 'NONE', #5626 ) ;
#3286=CARTESIAN_POINT ( 'NONE',  ( 1.999999999999986233, 15.00000000000000355, -4.000000000000009770 ) ) ;
#3294=DIRECTION ( 'NONE',  ( 1.000000000000000000, 0.000000000000000000, 0.000000000000000000 ) ) ;
#3306=VECTOR ( 'NONE', #7514, 1000.000000000000000 ) ;
#3310=ORIENTED_EDGE ( 'NONE', *, *, #7726, .T. ) ;
#3319=ORIENTED_EDGE ( 'NONE', *, *, #8304, .T. ) ;
#3332=ORIENTED_EDGE ( 'NONE', *, *, #6482, .F. ) ;
#3339=CARTESIAN_POINT ( 'NONE',  ( 30.00000000000001066, 0.000000000000000000, -1.599999999999986766 ) ) ;
#3345=PRODUCT_DEFINITION ( 'UNKNOWN', '', #7192, #80 ) ;
#3346=DIRECTION ( 'NONE',  ( 1.000000000000000000, 0.000000000000000000, 0.000000000000000000 ) ) ;
#3350=DIRECTION ( 'NONE',  ( 0.000000000000000000, 1.000000000000000000, 0.000000000000000000 ) ) ;
#3358=EDGE_LOOP ( 'NONE', ( #302, #8772 ) ) ;
#3371=ORIENTED_EDGE ( 'NONE', *, *, #6815, .F. ) ;
#3379=COLOUR_RGB ( '', 0.31764706, 0.68627451, 0.89019608) ;
#3384=VECTOR ( 'NONE', #331, 1000.000000000000000 ) ;
#3387=ORIENTED_EDGE ( 'NONE', *, *, #2650, .F. ) ;
#3415=FACE_OUTER_BOUND ( 'NONE', #8098, .T. ) ;
#3419=CARTESIAN_POINT ( 'NONE',  ( -26.99999999999998934, -13.00000000000000533, 0.000000000000000000 ) ) ;
#3420=EDGE_LOOP ( 'NONE', ( #5544, #3205, #3319, #6366 ) ) ;
#3425=LINE ( 'NONE', #6598, #4798 ) ;
#3427=EDGE_LOOP ( 'NONE', ( #9323, #8889 ) ) ;
#3443=CARTESIAN_POINT ( 'NONE',  ( 1.999999999999984901, 35.00000000000000000, 4.000000000000008882 ) ) ;
#3449=ORIENTED_EDGE ( 'NONE', *, *, #8054, .T. ) ;
#3452=ADVANCED_FACE ( 'NONE', ( #6680, #1717, #6633 ), #9939, .T. ) ;
#3455=MECHANICAL_DESIGN_GEOMETRIC_PRESENTATION_REPRESENTATION('',(#7856),#9558);
#3461=CARTESIAN_POINT ( 'NONE',  ( -15.00000000000000000, 19.99999999999999645, -9.000000000000000000 ) ) ;
#3479=AXIS2_PLACEMENT_3D ( 'NONE', #9861, #205, #5696 ) ;
#3486=EDGE_CURVE ( 'NONE', #409, #5519, #4096, .T. ) ;
#3493=EDGE_LOOP ( 'NONE', ( #1572, #7339, #5159, #1833 ) ) ;
#3509=EDGE_CURVE ( 'NONE', #9806, #8450, #8905, .T. ) ;
#3515=ORIENTED_EDGE ( 'NONE', *, *, #8588, .T. ) ;
#3518=DIRECTION ( 'NONE',  ( -1.000000000000000000, -4.625929269271485914E-16, 0.000000000000000000 ) ) ;
#3535=ORIENTED_EDGE ( 'NONE', *, *, #2362, .F. ) ;
#3539=DIRECTION ( 'NONE',  ( 0.000000000000000000, 0.000000000000000000, 1.000000000000000000 ) ) ;
#3540=VECTOR ( 'NONE', #9439, 1000.000000000000000 ) ;
#3549=ORIENTED_EDGE ( 'NONE', *, *, #5389, .T. ) ;
#3550=AXIS2_PLACEMENT_3D ( 'NONE', #2697, #9817, #4183 ) ;
#3551=FACE_OUTER_BOUND ( 'NONE', #4073, .T. ) ;
#3557=VECTOR ( 'NONE', #7890, 1000.000000000000000 ) ;
#3563=AXIS2_PLACEMENT_3D ( 'NONE', #9835, #373, #7576 ) ;
#3575=CIRCLE ( 'NONE', #7472, 2.000000000000003553 ) ;
#3580=ORIENTED_EDGE ( 'NONE', *, *, #6969, .F. ) ;
#3594=CARTESIAN_POINT ( 'NONE',  ( 27.00000000000001066, 0.000000000000000000, 0.000000000000000000 ) ) ;
#3601=ORIENTED_EDGE ( 'NONE', *, *, #8689, .F. ) ;
#3614=AXIS2_PLACEMENT_3D ( 'NONE', #5976, #2020, #8540 ) ;
#3627=ORIENTED_EDGE ( 'NONE', *, *, #3901, .F. ) ;
#3634=ORIENTED_EDGE ( 'NONE', *, *, #2488, .T. ) ;
#3641=VERTEX_POINT ( 'NONE', #4505 ) ;
#3644=VECTOR ( 'NONE', #2685, 1000.000000000000000 ) ;
#3663=CYLINDRICAL_SURFACE ( 'NONE', #7081, 1.249999999999993339 ) ;
#3669=LINE ( 'NONE', #6897, #5923 ) ;
#3682=EDGE_LOOP ( 'NONE', ( #6964, #6760, #4126, #6389 ) ) ;
#3690=VERTEX_POINT ( 'NONE', #2130 ) ;
#3695=LINE ( 'NONE', #9488, #5740 ) ;
#3696=EDGE_LOOP ( 'NONE', ( #4496, #4897, #8364, #8835 ) ) ;
#3705=DIRECTION ( 'NONE',  ( 0.000000000000000000, -0.000000000000000000, 1.000000000000000000 ) ) ;
#3706=ADVANCED_FACE ( 'NONE', ( #636, #8696 ), #7959, .T. ) ;
#3737=LINE ( 'NONE', #6966, #4741 ) ;
#3746=ORIENTED_EDGE ( 'NONE', *, *, #3043, .F. ) ;
#3763=DIRECTION ( 'NONE',  ( 1.000000000000000000, 0.000000000000000000, 0.000000000000000000 ) ) ;
#3765=ADVANCED_FACE ( 'NONE', ( #8750 ), #6992, .T. ) ;
#3771=VECTOR ( 'NONE', #1440, 1000.000000000000000 ) ;
#3787=CARTESIAN_POINT ( 'NONE',  ( -2.000000000000012879, 15.00000000000000355, 3.999999999999986233 ) ) ;
#3796=DIRECTION ( 'NONE',  ( 1.000000000000000000, 0.000000000000000000, 0.000000000000000000 ) ) ;
#3806=CARTESIAN_POINT ( 'NONE',  ( 1.999999999999986233, 15.00000000000000355, -4.000000000000009770 ) ) ;
#3814=DIRECTION ( 'NONE',  ( -0.000000000000000000, -0.000000000000000000, 1.000000000000000000 ) ) ;
#3822=CARTESIAN_POINT ( 'NONE',  ( 27.00000000000001066, -31.99999999999998579, 5.999999999999999112 ) ) ;
#3829=CARTESIAN_POINT ( 'NONE',  ( 1.999999999999984013, 35.00000000000000000, -4.000000000000009770 ) ) ;
#3834=FACE_OUTER_BOUND ( 'NONE', #2049, .T. ) ;
#3837=VERTEX_POINT ( 'NONE', #8015 ) ;
#3853=DIRECTION ( 'NONE',  ( -0.000000000000000000, -0.000000000000000000, -1.000000000000000000 ) ) ;
#3862=( NAMED_UNIT ( * ) SI_UNIT ( $, .STERADIAN. ) SOLID_ANGLE_UNIT ( ) );
#3867=DIRECTION ( 'NONE',  ( 0.000000000000000000, 0.000000000000000000, -1.000000000000000000 ) ) ;
#3878=CARTESIAN_POINT ( 'NONE',  ( -29.99999999999998934, 1.959434878635763751E-16, -1.599999999999998979 ) ) ;
#3883=CLOSED_SHELL ( 'NONE', ( #3962, #1480, #4190, #4420, #8088, #7341, #9148, #4823, #4397, #9846, #973, #4623, #3248, #9416, #6165, #10025, #7203, #3706, #3452, #10296, #7401, #1302, #1314, #7176, #3765, #2442, #2348, #1103, #4955, #7660, #7432, #7926, #1555, #8259, #6629, #530, #8863, #8841 ) ) ;
#3894=AXIS2_PLACEMENT_3D ( 'NONE', #2422, #5639, #4849 ) ;
#3899=DIRECTION ( 'NONE',  ( 1.000000000000000000, 0.000000000000000000, 0.000000000000000000 ) ) ;
#3901=EDGE_CURVE ( 'NONE', #9850, #5808, #4824, .T. ) ;
#3905=AXIS2_PLACEMENT_3D ( 'NONE', #38, #7395, #1829 ) ;
#3906=ORIENTED_EDGE ( 'NONE', *, *, #2662, .T. ) ;
#3909=DIRECTION ( 'NONE',  ( 0.000000000000000000, -0.000000000000000000, 1.000000000000000000 ) ) ;
#3912=EDGE_LOOP ( 'NONE', ( #1502, #8338, #322, #622 ) ) ;
#3916=ORIENTED_EDGE ( 'NONE', *, *, #5944, .T. ) ;
#3920=PRESENTATION_STYLE_ASSIGNMENT (( #688 ) ) ;
#3921=EDGE_LOOP ( 'NONE', ( #8999, #7146 ) ) ;
#3922=AXIS2_PLACEMENT_3D ( 'NONE', #8595, #3763, #3867 ) ;
#3923=LINE ( 'NONE', #692, #8385 ) ;
#3926=CARTESIAN_POINT ( 'NONE',  ( -2.000000000000024425, 15.00000000000000355, -5.999999999999988454 ) ) ;
#3929=LINE ( 'NONE', #6465, #5262 ) ;
#3934=DIRECTION ( 'NONE',  ( -1.000000000000000000, -1.156482317317871478E-16, 5.204170427930421283E-15 ) ) ;
#3938=CARTESIAN_POINT ( 'NONE',  ( 12.99999999999999645, 19.99999999999999645, -9.000000000000000000 ) ) ;
#3944=AXIS2_PLACEMENT_3D ( 'NONE', #9730, #2462, #5677 ) ;
#3946=VERTEX_POINT ( 'NONE', #3339 ) ;
#3947=VERTEX_POINT ( 'NONE', #1601 ) ;
#3962=ADVANCED_FACE ( 'NONE', ( #2499 ), #5712, .F. ) ;
#3965=CARTESIAN_POINT ( 'NONE',  ( -26.99999999999998934, 0.000000000000000000, 0.000000000000000000 ) ) ;
#3973=CARTESIAN_POINT ( 'NONE',  ( 30.00000000000001066, -34.99999999999999289, 9.000000000000000000 ) ) ;
#3978=DIRECTION ( 'NONE',  ( 1.000000000000000000, 0.000000000000000000, 0.000000000000000000 ) ) ;
#3996=CARTESIAN_POINT ( 'NONE',  ( 30.00000000000001066, -25.00000000000000000, 0.000000000000000000 ) ) ;
#4010=ORIENTED_EDGE ( 'NONE', *, *, #2543, .T. ) ;
#4038=CARTESIAN_POINT ( 'NONE',  ( 27.00000000000001066, -31.99999999999998579, 9.000000000000000000 ) ) ;
#4045=LINE ( 'NONE', #9838, #10321 ) ;
#4046=LINE ( 'NONE', #714, #2384 ) ;
#4057=DIRECTION ( 'NONE',  ( 0.000000000000000000, -0.000000000000000000, 1.000000000000000000 ) ) ;
#4065=ORIENTED_EDGE ( 'NONE', *, *, #6093, .T. ) ;
#4066=CARTESIAN_POINT ( 'NONE',  ( 30.00000000000001066, 0.000000000000000000, -1.599999999999992983 ) ) ;
#4068=CARTESIAN_POINT ( 'NONE',  ( -29.99999999999998934, -13.00000000000000533, -1.249999999999987121 ) ) ;
#4073=EDGE_LOOP ( 'NONE', ( #10105, #8361, #5226, #8583 ) ) ;
#4084=EDGE_CURVE ( 'NONE', #3946, #7840, #4896, .T. ) ;
#4093=LINE ( 'NONE', #7327, #1360 ) ;
#4096=LINE ( 'NONE', #125, #2647 ) ;
#4102=FACE_OUTER_BOUND ( 'NONE', #7464, .T. ) ;
#4109=DIRECTION ( 'NONE',  ( 1.000000000000000000, 0.000000000000000000, 0.000000000000000000 ) ) ;
#4126=ORIENTED_EDGE ( 'NONE', *, *, #6482, .T. ) ;
#4127=LINE ( 'NONE', #7367, #9402 ) ;
#4153=LINE ( 'NONE', #975, #4285 ) ;
#4176=ORIENTED_EDGE ( 'NONE', *, *, #7488, .F. ) ;
#4183=DIRECTION ( 'NONE',  ( 1.000000000000000000, 0.000000000000000000, 0.000000000000000000 ) ) ;
#4190=ADVANCED_FACE ( 'NONE', ( #2806 ), #6878, .F. ) ;
#4194=DIRECTION ( 'NONE',  ( -1.000000000000000000, -4.625929269271485914E-16, 0.000000000000000000 ) ) ;
#4204=LINE ( 'NONE', #9094, #1890 ) ;
#4205=DIRECTION ( 'NONE',  ( 0.000000000000000000, 0.000000000000000000, -1.000000000000000000 ) ) ;
#4206=ORIENTED_EDGE ( 'NONE', *, *, #8101, .F. ) ;
#4218=DIRECTION ( 'NONE',  ( -1.156482317317871478E-16, 1.000000000000000000, 0.000000000000000000 ) ) ;
#4233=EDGE_CURVE ( 'NONE', #2939, #409, #10398, .T. ) ;
#4247=CARTESIAN_POINT ( 'NONE',  ( -26.99999999999998934, 34.99999999999999289, -5.999999999999999112 ) ) ;
#4262=CARTESIAN_POINT ( 'NONE',  ( -15.00000000000000000, 19.99999999999999645, -5.999999999999999112 ) ) ;
#4269=ORIENTED_EDGE ( 'NONE', *, *, #5645, .F. ) ;
#4285=VECTOR ( 'NONE', #5838, 1000.000000000000000 ) ;
#4288=EDGE_LOOP ( 'NONE', ( #8053, #3580, #7927, #5963 ) ) ;
#4294=CARTESIAN_POINT ( 'NONE',  ( 30.00000000000001066, 35.00000000000001421, -9.000000000000000000 ) ) ;
#4317=LINE ( 'NONE', #9517, #10436 ) ;
#4367=CARTESIAN_POINT ( 'NONE',  ( 27.00000000000001066, -25.00000000000000000, 0.000000000000000000 ) ) ;
#4390=VECTOR ( 'NONE', #2652, 1000.000000000000000 ) ;
#4394=CARTESIAN_POINT ( 'NONE',  ( 0.000000000000000000, 0.000000000000000000, -5.999999999999999112 ) ) ;
#4397=ADVANCED_FACE ( 'NONE', ( #4585 ), #9372, .F. ) ;
#4399=VECTOR ( 'NONE', #9448, 1000.000000000000000 ) ;
#4403=CIRCLE ( 'NONE', #7808, 1.249999999999993339 ) ;
#4419=EDGE_LOOP ( 'NONE', ( #1035, #7285 ) ) ;
#4420=ADVANCED_FACE ( 'NONE', ( #9535 ), #10385, .F. ) ;
#4430=ORIENTED_EDGE ( 'NONE', *, *, #9523, .T. ) ;
#4435=MANIFOLD_SOLID_BREP ( 'M3 Clearance Hole2', #3883 ) ;
#4436=DIRECTION ( 'NONE',  ( 0.000000000000000000, 1.000000000000000000, 0.000000000000000000 ) ) ;
#4457=( GEOMETRIC_REPRESENTATION_CONTEXT ( 3 ) GLOBAL_UNCERTAINTY_ASSIGNED_CONTEXT ( ( #4485 ) ) GLOBAL_UNIT_ASSIGNED_CONTEXT ( ( #2386, #3177, #3862 ) ) REPRESENTATION_CONTEXT ( 'NONE', 'WORKASPACE' ) );
#4459=ORIENTED_EDGE ( 'NONE', *, *, #9528, .F. ) ;
#4467=DIRECTION ( 'NONE',  ( 1.000000000000000000, 0.000000000000000000, 0.000000000000000000 ) ) ;
#4474=ORIENTED_EDGE ( 'NONE', *, *, #4782, .F. ) ;
#4475=FACE_OUTER_BOUND ( 'NONE', #4511, .T. ) ;
#4477=DIRECTION ( 'NONE',  ( -1.000000000000000000, -4.625929269271485914E-16, 0.000000000000000000 ) ) ;
#4483=EDGE_CURVE ( 'NONE', #9543, #3690, #6970, .T. ) ;
#4485=UNCERTAINTY_MEASURE_WITH_UNIT (LENGTH_MEASURE( 1.000000000000000082E-05 ), #2386, 'distance_accuracy_value', 'NONE');
#4488=DIRECTION ( 'NONE',  ( 1.000000000000000000, -0.000000000000000000, -0.000000000000000000 ) ) ;
#4496=ORIENTED_EDGE ( 'NONE', *, *, #353, .F. ) ;
#4499=CARTESIAN_POINT ( 'NONE',  ( 30.00000000000001066, 1.959434878635756602E-16, 1.599999999999992983 ) ) ;
#4502=CARTESIAN_POINT ( 'NONE',  ( -26.99999999999998934, 0.000000000000000000, 1.599999999999998979 ) ) ;
#4504=CARTESIAN_POINT ( 'NONE',  ( -15.00000000000000000, 19.99999999999999645, -9.000000000000000000 ) ) ;
#4505=CARTESIAN_POINT ( 'NONE',  ( -2.000000000000024425, 15.00000000000000355, -5.999999999999999112 ) ) ;
#4506=CARTESIAN_POINT ( 'NONE',  ( 2.500000000000007105, -28.99999999999999289, 0.000000000000000000 ) ) ;
#4511=EDGE_LOOP ( 'NONE', ( #4700, #772, #1733, #1141 ) ) ;
#4514=CARTESIAN_POINT ( 'NONE',  ( -29.99999999999998934, -35.00000000000000000, -9.000000000000000000 ) ) ;
#4517=PRODUCT ( 'main housing', 'main housing', '', ( #3087 ) ) ;
#4530=FILL_AREA_STYLE_COLOUR ( '', #3379 ) ;
#4536=DIRECTION ( 'NONE',  ( 0.000000000000000000, -0.000000000000000000, 1.000000000000000000 ) ) ;
#4547=DIRECTION ( 'NONE',  ( 1.000000000000000000, 0.000000000000000000, 0.000000000000000000 ) ) ;
#4553=PLANE ( 'NONE',  #7386 ) ;
#4577=VECTOR ( 'NONE', #9461, 1000.000000000000000 ) ;
#4585=FACE_OUTER_BOUND ( 'NONE', #5910, .T. ) ;
#4591=DIRECTION ( 'NONE',  ( -1.000000000000000000, 0.000000000000000000, 0.000000000000000000 ) ) ;
#4623=ADVANCED_FACE ( 'NONE', ( #4904, #1577, #887 ), #6594, .F. ) ;
#4627=ORIENTED_EDGE ( 'NONE', *, *, #6480, .F. ) ;
#4629=DIRECTION ( 'NONE',  ( 0.000000000000000000, 0.000000000000000000, -1.000000000000000000 ) ) ;
#4643=DIRECTION ( 'NONE',  ( 0.000000000000000000, 0.000000000000000000, -1.000000000000000000 ) ) ;
#4644=CARTESIAN_POINT ( 'NONE',  ( -26.99999999999998934, -35.00000000000000000, -6.000000000000000000 ) ) ;
#4656=AXIS2_PLACEMENT_3D ( 'NONE', #4367, #6808, #8516 ) ;
#4674=EDGE_CURVE ( 'NONE', #8221, #2939, #8457, .T. ) ;
#4682=EDGE_LOOP ( 'NONE', ( #7052, #1423 ) ) ;
#4689=DIRECTION ( 'NONE',  ( 0.000000000000000000, 0.000000000000000000, -1.000000000000000000 ) ) ;
#4700=ORIENTED_EDGE ( 'NONE', *, *, #6153, .F. ) ;
#4703=FILL_AREA_STYLE ('',( #8745 ) ) ;
#4708=DIRECTION ( 'NONE',  ( -2.312964634635742957E-16, 1.000000000000000000, 0.000000000000000000 ) ) ;
#4718=VERTEX_POINT ( 'NONE', #7658 ) ;
#4723=ORIENTED_EDGE ( 'NONE', *, *, #4782, .T. ) ;
#4733=VECTOR ( 'NONE', #1409, 1000.000000000000000 ) ;
#4740=CARTESIAN_POINT ( 'NONE',  ( -2.499999999999992895, -28.99999999999999289, 3.061616997868383634E-16 ) ) ;
#4741=VECTOR ( 'NONE', #4477, 1000.000000000000000 ) ;
#4747=EDGE_LOOP ( 'NONE', ( #3271, #10167, #10210, #6129 ) ) ;
#4752=VECTOR ( 'NONE', #137, 1000.000000000000000 ) ;
#4770=CYLINDRICAL_SURFACE ( 'NONE', #3550, 2.000000000000001776 ) ;
#4776=DIRECTION ( 'NONE',  ( 0.000000000000000000, 0.000000000000000000, -1.000000000000000000 ) ) ;
#4782=EDGE_CURVE ( 'NONE', #2528, #3281, #1398, .T. ) ;
#4798=VECTOR ( 'NONE', #8206, 1000.000000000000000 ) ;
#4807=DIRECTION ( 'NONE',  ( -1.000000000000000000, 0.000000000000000000, 0.000000000000000000 ) ) ;
#4823=ADVANCED_FACE ( 'NONE', ( #3834 ), #7061, .F. ) ;
#4824=LINE ( 'NONE', #3237, #8742 ) ;
#4839=VECTOR ( 'NONE', #6471, 1000.000000000000000 ) ;
#4848=CARTESIAN_POINT ( 'NONE',  ( 27.00000000000001066, 35.00000000000001421, 9.000000000000000000 ) ) ;
#4849=DIRECTION ( 'NONE',  ( -1.000000000000000000, -1.156482317317871478E-16, 0.000000000000000000 ) ) ;
#4873=CARTESIAN_POINT ( 'NONE',  ( 27.00000000000001066, -25.00000000000000000, -1.999999999999997780 ) ) ;
#4878=EDGE_LOOP ( 'NONE', ( #6710, #6755, #9644, #6646, #9151, #2524, #10217, #1367 ) ) ;
#4886=VECTOR ( 'NONE', #2237, 1000.000000000000000 ) ;
#4887=CARTESIAN_POINT ( 'NONE',  ( -29.99999999999998934, 0.000000000000000000, 0.000000000000000000 ) ) ;
#4896=CIRCLE ( 'NONE', #7442, 1.599999999999986766 ) ;
#4897=ORIENTED_EDGE ( 'NONE', *, *, #6153, .T. ) ;
#4900=CARTESIAN_POINT ( 'NONE',  ( 1.999999999999975797, 15.00000000000000355, -6.000000000000009770 ) ) ;
#4904=FACE_BOUND ( 'NONE', #8942, .T. ) ;
#4905=VERTEX_POINT ( 'NONE', #8085 ) ;
#4909=ORIENTED_EDGE ( 'NONE', *, *, #8588, .F. ) ;
#4919=VERTEX_POINT ( 'NONE', #1566 ) ;
#4949=DIRECTION ( 'NONE',  ( 0.000000000000000000, 0.000000000000000000, 1.000000000000000000 ) ) ;
#4952=LINE ( 'NONE', #5106, #10029 ) ;
#4955=ADVANCED_FACE ( 'NONE', ( #4102 ), #9687, .T. ) ;
#4956=FACE_OUTER_BOUND ( 'NONE', #4747, .T. ) ;
#4958=ORIENTED_EDGE ( 'NONE', *, *, #10066, .F. ) ;
#4985=CARTESIAN_POINT ( 'NONE',  ( 30.00000000000001066, -25.00000000000000000, 0.000000000000000000 ) ) ;
#4995=DIRECTION ( 'NONE',  ( 1.000000000000000000, 2.312964634635742957E-16, 0.000000000000000000 ) ) ;
#5000=CIRCLE ( 'NONE', #2635, 1.599999999999998979 ) ;
#5004=EDGE_CURVE ( 'NONE', #7675, #4718, #4046, .T. ) ;
#5007=CARTESIAN_POINT ( 'NONE',  ( -2.000000000000015099, 35.00000000000000000, 3.999999999999986233 ) ) ;
#5009=CARTESIAN_POINT ( 'NONE',  ( 27.00000000000001066, -25.00000000000000000, 1.999999999999997780 ) ) ;
#5020=CARTESIAN_POINT ( 'NONE',  ( 1.999999999999987121, 15.00000000000000355, 4.000000000000008882 ) ) ;
#5021=CARTESIAN_POINT ( 'NONE',  ( 1.999999999999987121, 15.00000000000000355, 4.000000000000008882 ) ) ;
#5026=ORIENTED_EDGE ( 'NONE', *, *, #6178, .F. ) ;
#5037=DIRECTION ( 'NONE',  ( -1.000000000000000000, -0.000000000000000000, -0.000000000000000000 ) ) ;
#5039=DIRECTION ( 'NONE',  ( 1.000000000000000000, 0.000000000000000000, -0.000000000000000000 ) ) ;
#5041=DIRECTION ( 'NONE',  ( 0.000000000000000000, 0.000000000000000000, -1.000000000000000000 ) ) ;
#5066=ORIENTED_EDGE ( 'NONE', *, *, #2948, .F. ) ;
#5072=EDGE_CURVE ( 'NONE', #1747, #9420, #7149, .T. ) ;
#5074=AXIS2_PLACEMENT_3D ( 'NONE', #159, #9221, #5816 ) ;
#5090=CARTESIAN_POINT ( 'NONE',  ( 15.00000000000000000, 19.99999999999999645, -5.999999999999999112 ) ) ;
#5099=DIRECTION ( 'NONE',  ( -0.000000000000000000, -0.000000000000000000, 1.000000000000000000 ) ) ;
#5106=CARTESIAN_POINT ( 'NONE',  ( 30.00000000000001066, 35.00000000000001421, 9.000000000000000000 ) ) ;
#5109=VERTEX_POINT ( 'NONE', #2335 ) ;
#5116=VERTEX_POINT ( 'NONE', #5558 ) ;
#5131=CARTESIAN_POINT ( 'NONE',  ( 1.999999999999980904, 35.00000000000000000, -6.000000000000000000 ) ) ;
#5135=VECTOR ( 'NONE', #9025, 1000.000000000000000 ) ;
#5142=COLOUR_RGB ( '', 0.31764706, 0.68627451, 0.89019608) ;
#5153=EDGE_LOOP ( 'NONE', ( #10216, #10447 ) ) ;
#5159=ORIENTED_EDGE ( 'NONE', *, *, #447, .T. ) ;
#5170=CYLINDRICAL_SURFACE ( 'NONE', #8812, 2.500000000000000000 ) ;
#5185=CARTESIAN_POINT ( 'NONE',  ( -29.99999999999998934, -13.00000000000000533, 0.000000000000000000 ) ) ;
#5194=DIRECTION ( 'NONE',  ( -1.000000000000000000, -0.000000000000000000, -0.000000000000000000 ) ) ;
#5218=PLANE ( 'NONE',  #9856 ) ;
#5226=ORIENTED_EDGE ( 'NONE', *, *, #541, .T. ) ;
#5231=AXIS2_PLACEMENT_3D ( 'NONE', #778, #8886, #6593 ) ;
#5243=AXIS2_PLACEMENT_3D ( 'NONE', #2336, #635, #2497 ) ;
#5244=CYLINDRICAL_SURFACE ( 'NONE', #6777, 1.599999999999998979 ) ;
#5247=DIRECTION ( 'NONE',  ( 0.000000000000000000, 0.000000000000000000, 1.000000000000000000 ) ) ;
#5262=VECTOR ( 'NONE', #2555, 1000.000000000000000 ) ;
#5275=ORIENTED_EDGE ( 'NONE', *, *, #9516, .T. ) ;
#5287=ORIENTED_EDGE ( 'NONE', *, *, #2662, .F. ) ;
#5302=AXIS2_PLACEMENT_3D ( 'NONE', #9604, #1375, #2331 ) ;
#5303=FACE_OUTER_BOUND ( 'NONE', #1413, .T. ) ;
#5305=DIRECTION ( 'NONE',  ( 0.000000000000000000, 0.000000000000000000, 1.000000000000000000 ) ) ;
#5309=CIRCLE ( 'NONE', #9044, 1.249999999999987121 ) ;
#5317=ORIENTED_EDGE ( 'NONE', *, *, #1708, .T. ) ;
#5326=LINE ( 'NONE', #8612, #701 ) ;
#5328=DIRECTION ( 'NONE',  ( 1.156482317317871478E-16, -1.000000000000000000, -0.000000000000000000 ) ) ;
#5338=DIRECTION ( 'NONE',  ( 1.000000000000000000, 0.000000000000000000, -0.000000000000000000 ) ) ;
#5357=EDGE_CURVE ( 'NONE', #5372, #6021, #3669, .T. ) ;
#5360=ORIENTED_EDGE ( 'NONE', *, *, #5004, .F. ) ;
#5367=PLANE ( 'NONE',  #2533 ) ;
#5372=VERTEX_POINT ( 'NONE', #3141 ) ;
#5373=DIRECTION ( 'NONE',  ( -1.000000000000000000, -1.156482317317871478E-16, -5.637851296924623057E-15 ) ) ;
#5375=ORIENTED_EDGE ( 'NONE', *, *, #6053, .T. ) ;
#5379=CARTESIAN_POINT ( 'NONE',  ( 15.00000000000000000, 19.99999999999999645, -9.000000000000000000 ) ) ;
#5389=EDGE_CURVE ( 'NONE', #2210, #6021, #4093, .T. ) ;
#5400=DIRECTION ( 'NONE',  ( 1.000000000000000000, 0.000000000000000000, 0.000000000000000000 ) ) ;
#5428=CIRCLE ( 'NONE', #7642, 2.500000000000000000 ) ;
#5431=LINE ( 'NONE', #7236, #5927 ) ;
#5441=CARTESIAN_POINT ( 'NONE',  ( 1.999999999999973577, 35.00000000000000000, 6.000000000000010658 ) ) ;
#5443=ORIENTED_EDGE ( 'NONE', *, *, #6684, .T. ) ;
#5485=SURFACE_STYLE_FILL_AREA ( #6173 ) ;
#5519=VERTEX_POINT ( 'NONE', #6193 ) ;
#5533=EDGE_LOOP ( 'NONE', ( #8408, #5567, #10084, #3154 ) ) ;
#5544=ORIENTED_EDGE ( 'NONE', *, *, #1069, .F. ) ;
#5546=DIRECTION ( 'NONE',  ( -1.156482317317871478E-16, 1.000000000000000000, 0.000000000000000000 ) ) ;
#5554=CARTESIAN_POINT ( 'NONE',  ( 2.500000000000007550, -31.99999999999999289, 0.000000000000000000 ) ) ;
#5558=CARTESIAN_POINT ( 'NONE',  ( 12.99999999999999645, 19.99999999999999645, 9.000000000000000000 ) ) ;
#5567=ORIENTED_EDGE ( 'NONE', *, *, #9331, .F. ) ;
#5573=FACE_OUTER_BOUND ( 'NONE', #8154, .T. ) ;
#5594=CARTESIAN_POINT ( 'NONE',  ( 1.999999999999975797, 15.00000000000000355, -6.000000000000009770 ) ) ;
#5600=ORIENTED_EDGE ( 'NONE', *, *, #1579, .F. ) ;
#5610=DIRECTION ( 'NONE',  ( 0.000000000000000000, 0.000000000000000000, 1.000000000000000000 ) ) ;
#5611=ORIENTED_EDGE ( 'NONE', *, *, #6737, .T. ) ;
#5614=CYLINDRICAL_SURFACE ( 'NONE', #5243, 2.000000000000000000 ) ;
#5626=CARTESIAN_POINT ( 'NONE',  ( -13.00000000000000000, 19.99999999999999645, -5.999999999999999112 ) ) ;
#5636=VERTEX_POINT ( 'NONE', #4502 ) ;
#5639=DIRECTION ( 'NONE',  ( -1.156482317317871478E-16, 1.000000000000000000, 0.000000000000000000 ) ) ;
#5645=EDGE_CURVE ( 'NONE', #3690, #2579, #3923, .T. ) ;
#5653=EDGE_LOOP ( 'NONE', ( #9043, #1474, #724, #880 ) ) ;
#5660=ORIENTED_EDGE ( 'NONE', *, *, #8829, .F. ) ;
#5671=VECTOR ( 'NONE', #6604, 1000.000000000000000 ) ;
#5677=DIRECTION ( 'NONE',  ( -1.000000000000000000, 0.000000000000000000, 0.000000000000000000 ) ) ;
#5696=DIRECTION ( 'NONE',  ( -1.000000000000000000, 0.000000000000000000, 0.000000000000000000 ) ) ;
#5699=ORIENTED_EDGE ( 'NONE', *, *, #7412, .T. ) ;
#5706=EDGE_LOOP ( 'NONE', ( #1313, #6414 ) ) ;
#5712=CYLINDRICAL_SURFACE ( 'NONE', #6746, 1.599999999999992983 ) ;
#5721=CARTESIAN_POINT ( 'NONE',  ( 12.99999999999999645, 19.99999999999999645, 6.000000000000000000 ) ) ;
#5723=VECTOR ( 'NONE', #7214, 1000.000000000000000 ) ;
#5724=DIRECTION ( 'NONE',  ( 0.000000000000000000, 0.000000000000000000, 1.000000000000000000 ) ) ;
#5729=DIRECTION ( 'NONE',  ( -1.000000000000000000, 0.000000000000000000, 0.000000000000000000 ) ) ;
#5740=VECTOR ( 'NONE', #4436, 1000.000000000000000 ) ;
#5743=ORIENTED_EDGE ( 'NONE', *, *, #7899, .F. ) ;
#5746=LINE ( 'NONE', #7202, #8528 ) ;
#5752=PLANE ( 'NONE',  #9495 ) ;
#5763=VECTOR ( 'NONE', #9070, 1000.000000000000000 ) ;
#5766=CARTESIAN_POINT ( 'NONE',  ( 7.401486830834375884E-15, -31.99999999999999289, 0.000000000000000000 ) ) ;
#5785=DIRECTION ( 'NONE',  ( 0.000000000000000000, 0.000000000000000000, 1.000000000000000000 ) ) ;
#5798=ORIENTED_EDGE ( 'NONE', *, *, #3486, .T. ) ;
#5801=CIRCLE ( 'NONE', #5302, 2.000000000000000000 ) ;
#5808=VERTEX_POINT ( 'NONE', #8907 ) ;
#5816=DIRECTION ( 'NONE',  ( -5.694029147589358720E-15, 0.000000000000000000, 1.000000000000000000 ) ) ;
#5838=DIRECTION ( 'NONE',  ( 1.000000000000000000, 2.312964634635742957E-16, 0.000000000000000000 ) ) ;
#5839=ORIENTED_EDGE ( 'NONE', *, *, #1197, .T. ) ;
#5845=VECTOR ( 'NONE', #3518, 1000.000000000000000 ) ;
#5868=DIRECTION ( 'NONE',  ( -1.000000000000000000, -0.000000000000000000, -0.000000000000000000 ) ) ;
#5904=CARTESIAN_POINT ( 'NONE',  ( -26.99999999999998934, 1.959434878635763751E-16, -1.599999999999998979 ) ) ;
#5910=EDGE_LOOP ( 'NONE', ( #6952, #8554, #2502, #2811 ) ) ;
#5914=VECTOR ( 'NONE', #2883, 1000.000000000000000 ) ;
#5915=ORIENTED_EDGE ( 'NONE', *, *, #541, .F. ) ;
#5923=VECTOR ( 'NONE', #6102, 1000.000000000000000 ) ;
#5927=VECTOR ( 'NONE', #6273, 1000.000000000000000 ) ;
#5943=ORIENTED_EDGE ( 'NONE', *, *, #9694, .F. ) ;
#5944=EDGE_CURVE ( 'NONE', #9543, #5109, #4127, .T. ) ;
#5963=ORIENTED_EDGE ( 'NONE', *, *, #9940, .T. ) ;
#5965=LINE ( 'NONE', #3443, #4390 ) ;
#5975=DIRECTION ( 'NONE',  ( -1.000000000000000000, -2.312964634635742957E-16, 0.000000000000000000 ) ) ;
#5976=CARTESIAN_POINT ( 'NONE',  ( -15.00000000000000000, 19.99999999999999645, 9.000000000000000000 ) ) ;
#5980=DIRECTION ( 'NONE',  ( 0.000000000000000000, 0.000000000000000000, -1.000000000000000000 ) ) ;
#6000=ORIENTED_EDGE ( 'NONE', *, *, #7626, .F. ) ;
#6013=AXIS2_PLACEMENT_3D ( 'NONE', #2022, #6032, #5400 ) ;
#6021=VERTEX_POINT ( 'NONE', #8479 ) ;
#6022=DIRECTION ( 'NONE',  ( 0.000000000000000000, 0.000000000000000000, 1.000000000000000000 ) ) ;
#6023=CARTESIAN_POINT ( 'NONE',  ( 15.00000000000000000, 19.99999999999999645, -9.000000000000000000 ) ) ;
#6030=CARTESIAN_POINT ( 'NONE',  ( -29.99999999999998934, -13.00000000000000533, 0.000000000000000000 ) ) ;
#6032=DIRECTION ( 'NONE',  ( 0.000000000000000000, 0.000000000000000000, 1.000000000000000000 ) ) ;
#6040=ORIENTED_EDGE ( 'NONE', *, *, #3124, .T. ) ;
#6043=DIRECTION ( 'NONE',  ( -1.156482317317871478E-16, 1.000000000000000000, 0.000000000000000000 ) ) ;
#6050=VERTEX_POINT ( 'NONE', #8429 ) ;
#6053=EDGE_CURVE ( 'NONE', #118, #3161, #1782, .T. ) ;
#6054=DIRECTION ( 'NONE',  ( 1.000000000000000000, 0.000000000000000000, 0.000000000000000000 ) ) ;
#6055=CARTESIAN_POINT ( 'NONE',  ( 1.999999999999975797, 15.00000000000000355, 6.000000000000010658 ) ) ;
#6090=VECTOR ( 'NONE', #1373, 1000.000000000000000 ) ;
#6093=EDGE_CURVE ( 'NONE', #525, #7355, #5000, .T. ) ;
#6096=AXIS2_PLACEMENT_3D ( 'NONE', #3286, #6511, #8171 ) ;
#6102=DIRECTION ( 'NONE',  ( 5.204170427930421283E-15, 6.018531076210112041E-31, 1.000000000000000000 ) ) ;
#6114=CARTESIAN_POINT ( 'NONE',  ( 17.00000000000000000, 19.99999999999999645, 6.000000000000000000 ) ) ;
#6127=CARTESIAN_POINT ( 'NONE',  ( 0.000000000000000000, 0.000000000000000000, 9.000000000000000000 ) ) ;
#6129=ORIENTED_EDGE ( 'NONE', *, *, #6252, .T. ) ;
#6133=ORIENTED_EDGE ( 'NONE', *, *, #7193, .F. ) ;
#6135=APPLICATION_CONTEXT ( 'automotive_design' ) ;
#6153=EDGE_CURVE ( 'NONE', #8450, #6050, #8530, .T. ) ;
#6160=CARTESIAN_POINT ( 'NONE',  ( -13.00000000000000000, 19.99999999999999645, -9.000000000000000000 ) ) ;
#6165=ADVANCED_FACE ( 'NONE', ( #6921, #6977, #2909 ), #2113, .T. ) ;
#6170=ORIENTED_EDGE ( 'NONE', *, *, #6969, .T. ) ;
#6173=FILL_AREA_STYLE ('',( #4530 ) ) ;
#6176=AXIS2_PLACEMENT_3D ( 'NONE', #6127, #4536, #5338 ) ;
#6178=EDGE_CURVE ( 'NONE', #4919, #8624, #2798, .T. ) ;
#6180=ORIENTED_EDGE ( 'NONE', *, *, #2488, .F. ) ;
#6183=EDGE_LOOP ( 'NONE', ( #4909, #8985 ) ) ;
#6193=CARTESIAN_POINT ( 'NONE',  ( 30.00000000000001066, 35.00000000000001421, -9.000000000000000000 ) ) ;
#6198=CARTESIAN_POINT ( 'NONE',  ( 30.00000000000001066, -34.99999999999999289, -9.000000000000000000 ) ) ;
#6229=CIRCLE ( 'NONE', #492, 1.599999999999998979 ) ;
#6239=CARTESIAN_POINT ( 'NONE',  ( 30.00000000000001066, -25.00000000000000000, -1.999999999999997780 ) ) ;
#6252=EDGE_CURVE ( 'NONE', #2034, #8221, #676, .T. ) ;
#6262=CIRCLE ( 'NONE', #7978, 1.249999999999993339 ) ;
#6273=DIRECTION ( 'NONE',  ( -1.000000000000000000, -0.000000000000000000, -0.000000000000000000 ) ) ;
#6274=EDGE_CURVE ( 'NONE', #3161, #118, #1790, .T. ) ;
#6280=ORIENTED_EDGE ( 'NONE', *, *, #1197, .F. ) ;
#6283=VERTEX_POINT ( 'NONE', #5441 ) ;
#6296=DIRECTION ( 'NONE',  ( -5.694029147589358720E-15, -6.585044023479645679E-31, 1.000000000000000000 ) ) ;
#6298=DIRECTION ( 'NONE',  ( -1.000000000000000000, -4.625929269271485914E-16, 0.000000000000000000 ) ) ;
#6326=EDGE_CURVE ( 'NONE', #9821, #9979, #7245, .T. ) ;
#6332=CARTESIAN_POINT ( 'NONE',  ( 15.00000000000000000, 19.99999999999999645, 9.000000000000000000 ) ) ;
#6365=CARTESIAN_POINT ( 'NONE',  ( 0.000000000000000000, 0.000000000000000000, -9.000000000000000000 ) ) ;
#6366=ORIENTED_EDGE ( 'NONE', *, *, #5072, .T. ) ;
#6389=ORIENTED_EDGE ( 'NONE', *, *, #10242, .T. ) ;
#6414=ORIENTED_EDGE ( 'NONE', *, *, #9804, .T. ) ;
#6416=CARTESIAN_POINT ( 'NONE',  ( 1.999999999999975797, 15.00000000000000355, -6.000000000000009770 ) ) ;
#6435=DIRECTION ( 'NONE',  ( 1.000000000000000000, 1.156482317317871478E-16, 5.637851296924623057E-15 ) ) ;
#6443=CIRCLE ( 'NONE', #8148, 1.999999999999997780 ) ;
#6464=ORIENTED_EDGE ( 'NONE', *, *, #3901, .T. ) ;
#6465=CARTESIAN_POINT ( 'NONE',  ( 1.999999999999975797, 15.00000000000000355, 6.000000000000010658 ) ) ;
#6468=EDGE_CURVE ( 'NONE', #8145, #9102, #2532, .T. ) ;
#6471=DIRECTION ( 'NONE',  ( 1.000000000000000000, 2.312964634635742957E-16, -0.000000000000000000 ) ) ;
#6480=EDGE_CURVE ( 'NONE', #118, #3946, #834, .T. ) ;
#6482=EDGE_CURVE ( 'NONE', #4905, #2444, #8264, .T. ) ;
#6485=DIRECTION ( 'NONE',  ( -0.000000000000000000, -0.000000000000000000, -1.000000000000000000 ) ) ;
#6488=ORIENTED_EDGE ( 'NONE', *, *, #233, .T. ) ;
#6493=EDGE_CURVE ( 'NONE', #9654, #2939, #6551, .T. ) ;
#6499=SHAPE_REPRESENTATION ( 'main housing', ( #2101 ), #4457 ) ;
#6504=ORIENTED_EDGE ( 'NONE', *, *, #8134, .F. ) ;
#6506=EDGE_CURVE ( 'NONE', #1459, #5116, #8392, .T. ) ;
#6511=DIRECTION ( 'NONE',  ( -5.204170427930421283E-15, -6.018531076210112917E-31, -1.000000000000000000 ) ) ;
#6538=VERTEX_POINT ( 'NONE', #9962 ) ;
#6551=LINE ( 'NONE', #9803, #6687 ) ;
#6560=( NAMED_UNIT ( * ) SI_UNIT ( $, .STERADIAN. ) SOLID_ANGLE_UNIT ( ) );
#6566=EDGE_CURVE ( 'NONE', #7403, #2210, #4317, .T. ) ;
#6579=CARTESIAN_POINT ( 'NONE',  ( 27.00000000000001066, 0.000000000000000000, -1.599999999999992983 ) ) ;
#6593=DIRECTION ( 'NONE',  ( 0.000000000000000000, 0.000000000000000000, -1.000000000000000000 ) ) ;
#6594=PLANE ( 'NONE',  #7783 ) ;
#6598=CARTESIAN_POINT ( 'NONE',  ( -2.000000000000013767, 15.00000000000000355, -3.999999999999988898 ) ) ;
#6604=DIRECTION ( 'NONE',  ( -5.694029147589358720E-15, -6.585044023479645679E-31, 1.000000000000000000 ) ) ;
#6622=VERTEX_POINT ( 'NONE', #6114 ) ;
#6629=ADVANCED_FACE ( 'NONE', ( #4475 ), #7612, .F. ) ;
#6632=LINE ( 'NONE', #2663, #781 ) ;
#6633=FACE_OUTER_BOUND ( 'NONE', #8311, .T. ) ;
#6638=CARTESIAN_POINT ( 'NONE',  ( 27.00000000000001066, -25.00000000000000000, -1.999999999999997780 ) ) ;
#6642=CARTESIAN_POINT ( 'NONE',  ( -17.00000000000000000, 19.99999999999999645, -9.000000000000000000 ) ) ;
#6646=ORIENTED_EDGE ( 'NONE', *, *, #3043, .T. ) ;
#6673=DIRECTION ( 'NONE',  ( 0.000000000000000000, 0.000000000000000000, 1.000000000000000000 ) ) ;
#6680=FACE_BOUND ( 'NONE', #4682, .T. ) ;
#6684=EDGE_CURVE ( 'NONE', #3281, #6538, #8235, .T. ) ;
#6687=VECTOR ( 'NONE', #1046, 1000.000000000000000 ) ;
#6692=LINE ( 'NONE', #5007, #199 ) ;
#6710=ORIENTED_EDGE ( 'NONE', *, *, #6887, .F. ) ;
#6712=ORIENTED_EDGE ( 'NONE', *, *, #6274, .T. ) ;
#6721=DIRECTION ( 'NONE',  ( 1.000000000000000000, 0.000000000000000000, -0.000000000000000000 ) ) ;
#6737=EDGE_CURVE ( 'NONE', #2034, #9654, #6860, .T. ) ;
#6741=EDGE_LOOP ( 'NONE', ( #8710, #5066 ) ) ;
#6746=AXIS2_PLACEMENT_3D ( 'NONE', #1701, #7259, #9874 ) ;
#6753=VECTOR ( 'NONE', #5546, 1000.000000000000000 ) ;
#6754=CARTESIAN_POINT ( 'NONE',  ( -26.99999999999998934, 0.000000000000000000, 0.000000000000000000 ) ) ;
#6755=ORIENTED_EDGE ( 'NONE', *, *, #3199, .F. ) ;
#6760=ORIENTED_EDGE ( 'NONE', *, *, #8400, .T. ) ;
#6762=AXIS2_PLACEMENT_3D ( 'NONE', #2840, #2053, #8520 ) ;
#6765=ORIENTED_EDGE ( 'NONE', *, *, #8426, .T. ) ;
#6766=CARTESIAN_POINT ( 'NONE',  ( -29.99999999999998934, 0.000000000000000000, 0.000000000000000000 ) ) ;
#6776=DIRECTION ( 'NONE',  ( 1.156482317317871478E-16, -1.000000000000000000, -0.000000000000000000 ) ) ;
#6777=AXIS2_PLACEMENT_3D ( 'NONE', #1009, #5037, #6673 ) ;
#6780=VECTOR ( 'NONE', #5373, 1000.000000000000000 ) ;
#6787=DIRECTION ( 'NONE',  ( 1.000000000000000000, 0.000000000000000000, 0.000000000000000000 ) ) ;
#6796=CARTESIAN_POINT ( 'NONE',  ( -15.00000000000000000, 19.99999999999999645, 9.000000000000000000 ) ) ;
#6798=EDGE_LOOP ( 'NONE', ( #8515, #5287, #6488, #4176, #10136, #105, #9634, #4010, #3746, #10150, #207, #7568 ) ) ;
#6808=DIRECTION ( 'NONE',  ( 1.000000000000000000, -0.000000000000000000, -0.000000000000000000 ) ) ;
#6815=EDGE_CURVE ( 'NONE', #9654, #9197, #8027, .T. ) ;
#6819=VERTEX_POINT ( 'NONE', #5721 ) ;
#6837=CARTESIAN_POINT ( 'NONE',  ( 27.00000000000001066, -31.99999999999998579, -5.999999999999999112 ) ) ;
#6860=LINE ( 'NONE', #9308, #2135 ) ;
#6878=CYLINDRICAL_SURFACE ( 'NONE', #8965, 1.249999999999993339 ) ;
#6879=DIRECTION ( 'NONE',  ( 1.000000000000000000, 0.000000000000000000, 0.000000000000000000 ) ) ;
#6887=EDGE_CURVE ( 'NONE', #2001, #7403, #9623, .T. ) ;
#6895=CARTESIAN_POINT ( 'NONE',  ( -26.99999999999998934, -13.00000000000000533, -1.249999999999993339 ) ) ;
#6897=CARTESIAN_POINT ( 'NONE',  ( -2.000000000000026645, 35.00000000000000000, -5.999999999999988454 ) ) ;
#6921=FACE_BOUND ( 'NONE', #10417, .T. ) ;
#6934=FACE_OUTER_BOUND ( 'NONE', #3090, .T. ) ;
#6948=AXIS2_PLACEMENT_3D ( 'NONE', #4887, #8187, #5724 ) ;
#6952=ORIENTED_EDGE ( 'NONE', *, *, #9804, .F. ) ;
#6956=CARTESIAN_POINT ( 'NONE',  ( 30.00000000000001066, 0.000000000000000000, 0.000000000000000000 ) ) ;
#6964=ORIENTED_EDGE ( 'NONE', *, *, #2847, .F. ) ;
#6965=DIRECTION ( 'NONE',  ( 5.204170427930421283E-15, 0.000000000000000000, 1.000000000000000000 ) ) ;
#6966=CARTESIAN_POINT ( 'NONE',  ( 30.00000000000001066, 35.00000000000001421, 9.000000000000000000 ) ) ;
#6969=EDGE_CURVE ( 'NONE', #9821, #3947, #6632, .T. ) ;
#6970=LINE ( 'NONE', #2209, #4733 ) ;
#6977=FACE_BOUND ( 'NONE', #3358, .T. ) ;
#6987=DIRECTION ( 'NONE',  ( 0.000000000000000000, 1.000000000000000000, 0.000000000000000000 ) ) ;
#6992=PLANE ( 'NONE',  #8912 ) ;
#7005=EDGE_CURVE ( 'NONE', #5519, #8221, #7429, .T. ) ;
#7006=DIRECTION ( 'NONE',  ( -0.000000000000000000, -0.000000000000000000, 1.000000000000000000 ) ) ;
#7015=CARTESIAN_POINT ( 'NONE',  ( -2.000000000000026645, 35.00000000000000000, 5.999999999999987566 ) ) ;
#7021=DIRECTION ( 'NONE',  ( 1.000000000000000000, -0.000000000000000000, -0.000000000000000000 ) ) ;
#7044=FACE_BOUND ( 'NONE', #6183, .T. ) ;
#7050=DIRECTION ( 'NONE',  ( 0.000000000000000000, -0.000000000000000000, 1.000000000000000000 ) ) ;
#7052=ORIENTED_EDGE ( 'NONE', *, *, #6053, .F. ) ;
#7060=LINE ( 'NONE', #10310, #8123 ) ;
#7061=CYLINDRICAL_SURFACE ( 'NONE', #9147, 2.000000000000000000 ) ;
#7066=ORIENTED_EDGE ( 'NONE', *, *, #2232, .T. ) ;
#7081=AXIS2_PLACEMENT_3D ( 'NONE', #10144, #2079, #5305 ) ;
#7083=ORIENTED_EDGE ( 'NONE', *, *, #3509, .T. ) ;
#7090=CARTESIAN_POINT ( 'NONE',  ( 0.000000000000000000, 0.000000000000000000, 0.000000000000000000 ) ) ;
#7105=AXIS2_PLACEMENT_3D ( 'NONE', #10220, #1252, #7724 ) ;
#7110=DIRECTION ( 'NONE',  ( -1.000000000000000000, -0.000000000000000000, -0.000000000000000000 ) ) ;
#7112=LINE ( 'NONE', #10370, #522 ) ;
#7146=ORIENTED_EDGE ( 'NONE', *, *, #7412, .F. ) ;
#7149=LINE ( 'NONE', #10408, #4399 ) ;
#7150=LINE ( 'NONE', #3078, #8972 ) ;
#7158=FACE_BOUND ( 'NONE', #4419, .T. ) ;
#7159=ORIENTED_EDGE ( 'NONE', *, *, #9703, .T. ) ;
#7176=ADVANCED_FACE ( 'NONE', ( #5303 ), #1225, .F. ) ;
#7178=VECTOR ( 'NONE', #6987, 1000.000000000000000 ) ;
#7180=LINE ( 'NONE', #3787, #3225 ) ;
#7192=PRODUCT_DEFINITION_FORMATION_WITH_SPECIFIED_SOURCE ( 'ANY', '', #4517, .NOT_KNOWN. ) ;
#7193=EDGE_CURVE ( 'NONE', #2528, #8329, #1973, .T. ) ;
#7194=DIRECTION ( 'NONE',  ( 1.000000000000000000, 0.000000000000000000, 0.000000000000000000 ) ) ;
#7202=CARTESIAN_POINT ( 'NONE',  ( 17.00000000000000000, 19.99999999999999645, -9.000000000000000000 ) ) ;
#7203=ADVANCED_FACE ( 'NONE', ( #10244, #7044, #8593 ), #4553, .T. ) ;
#7214=DIRECTION ( 'NONE',  ( 1.156482317317871478E-16, -1.000000000000000000, -0.000000000000000000 ) ) ;
#7227=DIRECTION ( 'NONE',  ( 1.000000000000000000, 0.000000000000000000, 0.000000000000000000 ) ) ;
#7236=CARTESIAN_POINT ( 'NONE',  ( -29.99999999999998934, 0.000000000000000000, 1.599999999999998979 ) ) ;
#7237=PLANE ( 'NONE',  #3894 ) ;
#7245=LINE ( 'NONE', #2321, #1955 ) ;
#7257=DIRECTION ( 'NONE',  ( 1.000000000000000000, -0.000000000000000000, -0.000000000000000000 ) ) ;
#7259=DIRECTION ( 'NONE',  ( 1.000000000000000000, -0.000000000000000000, -0.000000000000000000 ) ) ;
#7272=AXIS2_PLACEMENT_3D ( 'NONE', #10231, #2804, #7684 ) ;
#7285=ORIENTED_EDGE ( 'NONE', *, *, #9528, .T. ) ;
#7294=DIRECTION ( 'NONE',  ( 1.000000000000000000, 0.000000000000000000, -0.000000000000000000 ) ) ;
#7308=CARTESIAN_POINT ( 'NONE',  ( 30.00000000000001066, -34.99999999999999289, 9.000000000000000000 ) ) ;
#7310=ORIENTED_EDGE ( 'NONE', *, *, #6326, .F. ) ;
#7316=EDGE_CURVE ( 'NONE', #2753, #7403, #7150, .T. ) ;
#7317=FACE_OUTER_BOUND ( 'NONE', #565, .T. ) ;
#7327=CARTESIAN_POINT ( 'NONE',  ( 1.999999999999984013, 35.00000000000000000, -4.000000000000009770 ) ) ;
#7330=CYLINDRICAL_SURFACE ( 'NONE', #3563, 1.599999999999992983 ) ;
#7339=ORIENTED_EDGE ( 'NONE', *, *, #10201, .F. ) ;
#7341=ADVANCED_FACE ( 'NONE', ( #2393 ), #5614, .F. ) ;
#7342=ORIENTED_EDGE ( 'NONE', *, *, #7005, .T. ) ;
#7355=VERTEX_POINT ( 'NONE', #2284 ) ;
#7367=CARTESIAN_POINT ( 'NONE',  ( -2.000000000000012879, 15.00000000000000355, 3.999999999999986233 ) ) ;
#7386=AXIS2_PLACEMENT_3D ( 'NONE', #7800, #536, #9449 ) ;
#7387=DIRECTION ( 'NONE',  ( 0.000000000000000000, -1.000000000000000000, -0.000000000000000000 ) ) ;
#7395=DIRECTION ( 'NONE',  ( -1.156482317317871478E-16, 1.000000000000000000, 0.000000000000000000 ) ) ;
#7401=ADVANCED_FACE ( 'NONE', ( #746 ), #4770, .F. ) ;
#7403=VERTEX_POINT ( 'NONE', #5131 ) ;
#7407=ORIENTED_EDGE ( 'NONE', *, *, #10201, .T. ) ;
#7412=EDGE_CURVE ( 'NONE', #1211, #9529, #1014, .T. ) ;
#7417=DIRECTION ( 'NONE',  ( -1.000000000000000000, 0.000000000000000000, 0.000000000000000000 ) ) ;
#7429=LINE ( 'NONE', #4294, #8406 ) ;
#7432=ADVANCED_FACE ( 'NONE', ( #7479 ), #2548, .F. ) ;
#7442=AXIS2_PLACEMENT_3D ( 'NONE', #2654, #9223, #7630 ) ;
#7464=EDGE_LOOP ( 'NONE', ( #4269, #2387, #3916, #3310 ) ) ;
#7472=AXIS2_PLACEMENT_3D ( 'NONE', #6332, #3162, #1524 ) ;
#7478=CARTESIAN_POINT ( 'NONE',  ( -29.99999999999998934, -13.00000000000000533, 1.249999999999987121 ) ) ;
#7479=FACE_OUTER_BOUND ( 'NONE', #2319, .T. ) ;
#7485=FACE_OUTER_BOUND ( 'NONE', #3011, .T. ) ;
#7488=EDGE_CURVE ( 'NONE', #48, #6283, #5965, .T. ) ;
#7496=CARTESIAN_POINT ( 'NONE',  ( -17.00000000000000000, 19.99999999999999645, 6.000000000000000000 ) ) ;
#7502=ORIENTED_EDGE ( 'NONE', *, *, #353, .T. ) ;
#7504=VECTOR ( 'NONE', #681, 1000.000000000000000 ) ;
#7512=ORIENTED_EDGE ( 'NONE', *, *, #2543, .F. ) ;
#7514=DIRECTION ( 'NONE',  ( -1.000000000000000000, -0.000000000000000000, -0.000000000000000000 ) ) ;
#7519=ORIENTED_EDGE ( 'NONE', *, *, #1377, .F. ) ;
#7525=ORIENTED_EDGE ( 'NONE', *, *, #8186, .T. ) ;
#7559=EDGE_LOOP ( 'NONE', ( #2521, #8746 ) ) ;
#7562=CARTESIAN_POINT ( 'NONE',  ( -15.00000000000000000, 19.99999999999999645, -5.999999999999999112 ) ) ;
#7563=FACE_OUTER_BOUND ( 'NONE', #805, .T. ) ;
#7568=ORIENTED_EDGE ( 'NONE', *, *, #6566, .F. ) ;
#7576=DIRECTION ( 'NONE',  ( 0.000000000000000000, 0.000000000000000000, -1.000000000000000000 ) ) ;
#7579=EDGE_LOOP ( 'NONE', ( #1196, #5660 ) ) ;
#7612=CYLINDRICAL_SURFACE ( 'NONE', #4656, 1.999999999999997780 ) ;
#7626=EDGE_CURVE ( 'NONE', #317, #2753, #3695, .T. ) ;
#7630=DIRECTION ( 'NONE',  ( 0.000000000000000000, 0.000000000000000000, -1.000000000000000000 ) ) ;
#7640=VECTOR ( 'NONE', #7110, 1000.000000000000000 ) ;
#7642=AXIS2_PLACEMENT_3D ( 'NONE', #1612, #8433, #1964 ) ;
#7654=DIRECTION ( 'NONE',  ( 0.000000000000000000, 0.000000000000000000, 1.000000000000000000 ) ) ;
#7658=CARTESIAN_POINT ( 'NONE',  ( -13.00000000000000000, 19.99999999999999645, 9.000000000000000000 ) ) ;
#7660=ADVANCED_FACE ( 'NONE', ( #471 ), #10077, .F. ) ;
#7667=DIRECTION ( 'NONE',  ( 0.000000000000000000, -0.000000000000000000, 1.000000000000000000 ) ) ;
#7675=VERTEX_POINT ( 'NONE', #2961 ) ;
#7682=ORIENTED_EDGE ( 'NONE', *, *, #7488, .T. ) ;
#7684=DIRECTION ( 'NONE',  ( 1.000000000000000000, 0.000000000000000000, 5.637851296924623057E-15 ) ) ;
#7693=CARTESIAN_POINT ( 'NONE',  ( -2.000000000000013767, 15.00000000000000355, -3.999999999999988898 ) ) ;
#7702=DIRECTION ( 'NONE',  ( 1.000000000000000000, 0.000000000000000000, 0.000000000000000000 ) ) ;
#7705=AXIS2_PLACEMENT_3D ( 'NONE', #3594, #4591, #3539 ) ;
#7706=EDGE_LOOP ( 'NONE', ( #8559, #9090, #5699, #5915 ) ) ;
#7722=AXIS2_PLACEMENT_3D ( 'NONE', #8452, #6043, #8557 ) ;
#7724=DIRECTION ( 'NONE',  ( 1.000000000000000000, 0.000000000000000000, 0.000000000000000000 ) ) ;
#7726=EDGE_CURVE ( 'NONE', #5109, #2579, #570, .T. ) ;
#7728=EDGE_CURVE ( 'NONE', #9979, #10188, #3065, .T. ) ;
#7772=ORIENTED_EDGE ( 'NONE', *, *, #7853, .T. ) ;
#7775=SURFACE_STYLE_USAGE ( .BOTH. , #2157 ) ;
#7777=STYLED_ITEM ( 'NONE', ( #3058 ), #4435 ) ;
#7783=AXIS2_PLACEMENT_3D ( 'NONE', #2578, #4057, #7294 ) ;
#7789=ORIENTED_EDGE ( 'NONE', *, *, #8101, .T. ) ;
#7795=SURFACE_STYLE_FILL_AREA ( #4703 ) ;
#7800=CARTESIAN_POINT ( 'NONE',  ( -26.99999999999998934, -35.00000000000000000, 9.000000000000000000 ) ) ;
#7807=CIRCLE ( 'NONE', #1881, 2.000000000000000000 ) ;
#7808=AXIS2_PLACEMENT_3D ( 'NONE', #8354, #2778, #1185 ) ;
#7832=EDGE_LOOP ( 'NONE', ( #8990, #6180, #9269, #8830, #3113, #7310, #6280, #3601 ) ) ;
#7840=VERTEX_POINT ( 'NONE', #2270 ) ;
#7853=EDGE_CURVE ( 'NONE', #5636, #8002, #1875, .T. ) ;
#7856=STYLED_ITEM ( 'NONE', ( #3920 ), #8040 ) ;
#7878=VERTEX_POINT ( 'NONE', #4068 ) ;
#7890=DIRECTION ( 'NONE',  ( 0.000000000000000000, -1.000000000000000000, -0.000000000000000000 ) ) ;
#7899=EDGE_CURVE ( 'NONE', #292, #3947, #1418, .T. ) ;
#7917=LINE ( 'NONE', #3878, #7640 ) ;
#7926=ADVANCED_FACE ( 'NONE', ( #7563 ), #5752, .T. ) ;
#7927=ORIENTED_EDGE ( 'NONE', *, *, #6326, .T. ) ;
#7959=PLANE ( 'NONE',  #9252 ) ;
#7964=EDGE_CURVE ( 'NONE', #8145, #48, #9805, .T. ) ;
#7974=CARTESIAN_POINT ( 'NONE',  ( 30.00000000000001066, 35.00000000000001421, 9.000000000000000000 ) ) ;
#7978=AXIS2_PLACEMENT_3D ( 'NONE', #3419, #4109, #4205 ) ;
#7979=FACE_OUTER_BOUND ( 'NONE', #3420, .T. ) ;
#7989=LINE ( 'NONE', #4900, #4752 ) ;
#8002=VERTEX_POINT ( 'NONE', #5904 ) ;
#8015=CARTESIAN_POINT ( 'NONE',  ( 2.500000000000007105, -28.99999999999999289, 0.000000000000000000 ) ) ;
#8016=CIRCLE ( 'NONE', #3944, 2.000000000000003553 ) ;
#8023=ORIENTED_EDGE ( 'NONE', *, *, #10380, .F. ) ;
#8024=AXIS2_PLACEMENT_3D ( 'NONE', #4262, #8413, #1891 ) ;
#8027=LINE ( 'NONE', #8183, #4839 ) ;
#8029=CARTESIAN_POINT ( 'NONE',  ( -2.000000000000024425, 15.00000000000000355, -5.999999999999988454 ) ) ;
#8039=ORIENTED_EDGE ( 'NONE', *, *, #9694, .T. ) ;
#8040=ADVANCED_BREP_SHAPE_REPRESENTATION ( '', ( #4435, #2101 ), #4457 ) ;
#8053=ORIENTED_EDGE ( 'NONE', *, *, #9868, .F. ) ;
#8054=EDGE_CURVE ( 'NONE', #8002, #5636, #8635, .T. ) ;
#8069=CARTESIAN_POINT ( 'NONE',  ( -15.00000000000000000, 19.99999999999999645, 6.000000000000000000 ) ) ;
#8085=CARTESIAN_POINT ( 'NONE',  ( -26.99999999999998934, -13.00000000000000533, 1.249999999999993339 ) ) ;
#8088=ADVANCED_FACE ( 'NONE', ( #10166 ), #5170, .T. ) ;
#8098=EDGE_LOOP ( 'NONE', ( #5798, #269, #3173, #5275 ) ) ;
#8101=EDGE_CURVE ( 'NONE', #2891, #2034, #3737, .T. ) ;
#8103=ORIENTED_EDGE ( 'NONE', *, *, #5072, .F. ) ;
#8106=EDGE_LOOP ( 'NONE', ( #6765, #1132 ) ) ;
#8123=VECTOR ( 'NONE', #3044, 1000.000000000000000 ) ;
#8134=EDGE_CURVE ( 'NONE', #9850, #7675, #1702, .T. ) ;
#8135=DIRECTION ( 'NONE',  ( -1.000000000000000000, 0.000000000000000000, 0.000000000000000000 ) ) ;
#8137=ORIENTED_EDGE ( 'NONE', *, *, #8140, .F. ) ;
#8140=EDGE_CURVE ( 'NONE', #6819, #6622, #8476, .T. ) ;
#8145=VERTEX_POINT ( 'NONE', #2950 ) ;
#8148=AXIS2_PLACEMENT_3D ( 'NONE', #3996, #7227, #8604 ) ;
#8154=EDGE_LOOP ( 'NONE', ( #7342, #8838, #4206, #2896 ) ) ;
#8156=VECTOR ( 'NONE', #7257, 1000.000000000000000 ) ;
#8162=DIRECTION ( 'NONE',  ( 1.156482317317871478E-16, -1.000000000000000000, -0.000000000000000000 ) ) ;
#8171=DIRECTION ( 'NONE',  ( -1.000000000000000000, 0.000000000000000000, 5.204170427930421283E-15 ) ) ;
#8172=DIRECTION ( 'NONE',  ( -1.156482317317871478E-16, 1.000000000000000000, 0.000000000000000000 ) ) ;
#8183=CARTESIAN_POINT ( 'NONE',  ( 30.00000000000001066, -34.99999999999999289, 9.000000000000000000 ) ) ;
#8186=EDGE_CURVE ( 'NONE', #9543, #8145, #7180, .T. ) ;
#8187=DIRECTION ( 'NONE',  ( -1.000000000000000000, -0.000000000000000000, -0.000000000000000000 ) ) ;
#8194=CARTESIAN_POINT ( 'NONE',  ( -26.99999999999998934, -32.00000000000000000, 5.999999999999999112 ) ) ;
#8201=AXIS2_PLACEMENT_3D ( 'NONE', #2505, #68, #3346 ) ;
#8202=FACE_BOUND ( 'NONE', #3427, .T. ) ;
#8206=DIRECTION ( 'NONE',  ( -1.156482317317871478E-16, 1.000000000000000000, 0.000000000000000000 ) ) ;
#8207=ORIENTED_EDGE ( 'NONE', *, *, #6468, .F. ) ;
#8221=VERTEX_POINT ( 'NONE', #3002 ) ;
#8235=CIRCLE ( 'NONE', #9421, 2.000000000000000000 ) ;
#8239=VECTOR ( 'NONE', #3039, 1000.000000000000000 ) ;
#8259=ADVANCED_FACE ( 'NONE', ( #9472 ), #7237, .T. ) ;
#8264=LINE ( 'NONE', #990, #3306 ) ;
#8304=EDGE_CURVE ( 'NONE', #2001, #1747, #7989, .T. ) ;
#8311=EDGE_LOOP ( 'NONE', ( #6000, #9137, #659, #3906 ) ) ;
#8313=AXIS2_PLACEMENT_3D ( 'NONE', #6754, #9208, #1947 ) ;
#8329=VERTEX_POINT ( 'NONE', #6642 ) ;
#8338=ORIENTED_EDGE ( 'NONE', *, *, #7005, .F. ) ;
#8340=CARTESIAN_POINT ( 'NONE',  ( 30.00000000000001066, -34.99999999999999289, 9.000000000000000000 ) ) ;
#8351=EDGE_LOOP ( 'NONE', ( #5600, #6133, #4723, #5443 ) ) ;
#8354=CARTESIAN_POINT ( 'NONE',  ( -26.99999999999998934, -13.00000000000000533, 0.000000000000000000 ) ) ;
#8360=CARTESIAN_POINT ( 'NONE',  ( -29.99999999999998934, -35.00000000000000000, 9.000000000000000000 ) ) ;
#8361=ORIENTED_EDGE ( 'NONE', *, *, #8426, .F. ) ;
#8364=ORIENTED_EDGE ( 'NONE', *, *, #8829, .T. ) ;
#8385=VECTOR ( 'NONE', #6296, 1000.000000000000000 ) ;
#8392=CIRCLE ( 'NONE', #3479, 2.000000000000003553 ) ;
#8398=VECTOR ( 'NONE', #3853, 1000.000000000000000 ) ;
#8400=EDGE_CURVE ( 'NONE', #9902, #4905, #6262, .T. ) ;
#8402=AXIS2_PLACEMENT_3D ( 'NONE', #8975, #8135, #916 ) ;
#8405=DIRECTION ( 'NONE',  ( 1.000000000000000000, -0.000000000000000000, -0.000000000000000000 ) ) ;
#8406=VECTOR ( 'NONE', #4194, 1000.000000000000000 ) ;
#8408=ORIENTED_EDGE ( 'NONE', *, *, #5357, .F. ) ;
#8413=DIRECTION ( 'NONE',  ( 0.000000000000000000, -0.000000000000000000, 1.000000000000000000 ) ) ;
#8426=EDGE_CURVE ( 'NONE', #3837, #2653, #9501, .T. ) ;
#8429=CARTESIAN_POINT ( 'NONE',  ( 30.00000000000001066, -25.00000000000000000, 1.999999999999997780 ) ) ;
#8431=ORIENTED_EDGE ( 'NONE', *, *, #6480, .T. ) ;
#8433=DIRECTION ( 'NONE',  ( -1.156482317317871478E-16, 1.000000000000000000, 0.000000000000000000 ) ) ;
#8447=CYLINDRICAL_SURFACE ( 'NONE', #516, 2.000000000000001776 ) ;
#8450=VERTEX_POINT ( 'NONE', #5009 ) ;
#8452=CARTESIAN_POINT ( 'NONE',  ( 7.054542135639013677E-15, -28.99999999999999289, 0.000000000000000000 ) ) ;
#8457=LINE ( 'NONE', #1189, #341 ) ;
#8461=ORIENTED_EDGE ( 'NONE', *, *, #1708, .F. ) ;
#8474=EDGE_LOOP ( 'NONE', ( #5743, #7512, #5839, #6170 ) ) ;
#8476=CIRCLE ( 'NONE', #7105, 2.000000000000001776 ) ;
#8479=CARTESIAN_POINT ( 'NONE',  ( -2.000000000000015987, 35.00000000000000000, -3.999999999999988898 ) ) ;
#8496=CARTESIAN_POINT ( 'NONE',  ( -29.99999999999998934, 0.000000000000000000, 1.599999999999998979 ) ) ;
#8501=VERTEX_POINT ( 'NONE', #1934 ) ;
#8515=ORIENTED_EDGE ( 'NONE', *, *, #7316, .F. ) ;
#8516=DIRECTION ( 'NONE',  ( 0.000000000000000000, 0.000000000000000000, -1.000000000000000000 ) ) ;
#8517=CARTESIAN_POINT ( 'NONE',  ( 1.999999999999975797, 15.00000000000000355, -6.000000000000009770 ) ) ;
#8520=DIRECTION ( 'NONE',  ( 1.000000000000000000, 0.000000000000000000, 0.000000000000000000 ) ) ;
#8528=VECTOR ( 'NONE', #9904, 1000.000000000000000 ) ;
#8530=LINE ( 'NONE', #1262, #10091 ) ;
#8540=DIRECTION ( 'NONE',  ( 1.000000000000000000, 0.000000000000000000, 0.000000000000000000 ) ) ;
#8554=ORIENTED_EDGE ( 'NONE', *, *, #10126, .T. ) ;
#8557=DIRECTION ( 'NONE',  ( -1.000000000000000000, 0.000000000000000000, 0.000000000000000000 ) ) ;
#8559=ORIENTED_EDGE ( 'NONE', *, *, #3008, .F. ) ;
#8574=CARTESIAN_POINT ( 'NONE',  ( 27.00000000000001066, -25.00000000000000000, 0.000000000000000000 ) ) ;
#8575=EDGE_LOOP ( 'NONE', ( #8461, #6712, #8431, #10227 ) ) ;
#8583=ORIENTED_EDGE ( 'NONE', *, *, #8881, .T. ) ;
#8588=EDGE_CURVE ( 'NONE', #4905, #9902, #4403, .T. ) ;
#8591=PLANE ( 'NONE',  #921 ) ;
#8593=FACE_OUTER_BOUND ( 'NONE', #8474, .T. ) ;
#8595=CARTESIAN_POINT ( 'NONE',  ( 27.00000000000001066, -25.00000000000000000, 0.000000000000000000 ) ) ;
#8604=DIRECTION ( 'NONE',  ( 0.000000000000000000, 0.000000000000000000, -1.000000000000000000 ) ) ;
#8605=EDGE_LOOP ( 'NONE', ( #1948, #2740, #556, #92 ) ) ;
#8612=CARTESIAN_POINT ( 'NONE',  ( -26.99999999999998934, 34.99999999999999289, 9.000000000000000000 ) ) ;
#8618=( NAMED_UNIT ( * ) SI_UNIT ( $, .STERADIAN. ) SOLID_ANGLE_UNIT ( ) );
#8624=VERTEX_POINT ( 'NONE', #2144 ) ;
#8632=CARTESIAN_POINT ( 'NONE',  ( 1.999999999999987121, 15.00000000000000355, 5.999999999999999112 ) ) ;
#8635=CIRCLE ( 'NONE', #8313, 1.599999999999998979 ) ;
#8689=EDGE_CURVE ( 'NONE', #2579, #8501, #1395, .T. ) ;
#8696=FACE_OUTER_BOUND ( 'NONE', #4288, .T. ) ;
#8710=ORIENTED_EDGE ( 'NONE', *, *, #4084, .F. ) ;
#8724=( NAMED_UNIT ( * ) PLANE_ANGLE_UNIT ( ) SI_UNIT ( $, .RADIAN. ) );
#8742=VECTOR ( 'NONE', #221, 1000.000000000000000 ) ;
#8744=CARTESIAN_POINT ( 'NONE',  ( -2.000000000000012879, 15.00000000000000355, 3.999999999999986233 ) ) ;
#8745=FILL_AREA_STYLE_COLOUR ( '', #5142 ) ;
#8746=ORIENTED_EDGE ( 'NONE', *, *, #398, .F. ) ;
#8750=FACE_OUTER_BOUND ( 'NONE', #5533, .T. ) ;
#8772=ORIENTED_EDGE ( 'NONE', *, *, #1971, .F. ) ;
#8779=( LENGTH_UNIT ( ) NAMED_UNIT ( * ) SI_UNIT ( .MILLI., .METRE. ) );
#8812=AXIS2_PLACEMENT_3D ( 'NONE', #9310, #5328, #1201 ) ;
#8813=EDGE_CURVE ( 'NONE', #6819, #5116, #7112, .T. ) ;
#8821=DIRECTION ( 'NONE',  ( 1.000000000000000000, 4.625929269271485914E-16, 0.000000000000000000 ) ) ;
#8829=EDGE_CURVE ( 'NONE', #6050, #9585, #6443, .T. ) ;
#8830=ORIENTED_EDGE ( 'NONE', *, *, #233, .F. ) ;
#8835=ORIENTED_EDGE ( 'NONE', *, *, #2258, .F. ) ;
#8838=ORIENTED_EDGE ( 'NONE', *, *, #6252, .F. ) ;
#8841=ADVANCED_FACE ( 'NONE', ( #1337 ), #7330, .F. ) ;
#8855=DIRECTION ( 'NONE',  ( 0.000000000000000000, -0.000000000000000000, 1.000000000000000000 ) ) ;
#8859=AXIS2_PLACEMENT_3D ( 'NONE', #8340, #10040, #5975 ) ;
#8863=ADVANCED_FACE ( 'NONE', ( #9781 ), #870, .F. ) ;
#8867=AXIS2_PLACEMENT_3D ( 'NONE', #923, #9994, #5785 ) ;
#8881=EDGE_CURVE ( 'NONE', #9529, #1211, #5428, .T. ) ;
#8886=DIRECTION ( 'NONE',  ( 1.000000000000000000, 0.000000000000000000, 0.000000000000000000 ) ) ;
#8889=ORIENTED_EDGE ( 'NONE', *, *, #10256, .F. ) ;
#8905=CIRCLE ( 'NONE', #10264, 1.999999999999997780 ) ;
#8907=CARTESIAN_POINT ( 'NONE',  ( -17.00000000000000000, 19.99999999999999645, 9.000000000000000000 ) ) ;
#8908=PLANE ( 'NONE',  #6096 ) ;
#8912=AXIS2_PLACEMENT_3D ( 'NONE', #3926, #10245, #1432 ) ;
#8920=SHAPE_DEFINITION_REPRESENTATION ( #3179, #6499 ) ;
#8926=DIRECTION ( 'NONE',  ( -5.694029147589358720E-15, 0.000000000000000000, 1.000000000000000000 ) ) ;
#8936=EDGE_LOOP ( 'NONE', ( #6504, #6464, #2066, #5360 ) ) ;
#8942=EDGE_LOOP ( 'NONE', ( #7407, #2011 ) ) ;
#8953=EDGE_CURVE ( 'NONE', #9040, #3277, #8016, .T. ) ;
#8965=AXIS2_PLACEMENT_3D ( 'NONE', #5185, #5868, #6022 ) ;
#8972=VECTOR ( 'NONE', #6298, 1000.000000000000000 ) ;
#8975=CARTESIAN_POINT ( 'NONE',  ( 27.00000000000001066, -34.99999999999999289, 9.000000000000000000 ) ) ;
#8977=CARTESIAN_POINT ( 'NONE',  ( 1.999999999999984901, 35.00000000000000000, 4.000000000000008882 ) ) ;
#8984=FACE_BOUND ( 'NONE', #6741, .T. ) ;
#8985=ORIENTED_EDGE ( 'NONE', *, *, #8400, .F. ) ;
#8990=ORIENTED_EDGE ( 'NONE', *, *, #7726, .F. ) ;
#8992=VECTOR ( 'NONE', #9981, 1000.000000000000000 ) ;
#8999=ORIENTED_EDGE ( 'NONE', *, *, #8881, .F. ) ;
#9025=DIRECTION ( 'NONE',  ( -0.000000000000000000, -0.000000000000000000, 1.000000000000000000 ) ) ;
#9040=VERTEX_POINT ( 'NONE', #2965 ) ;
#9043=ORIENTED_EDGE ( 'NONE', *, *, #2803, .T. ) ;
#9044=AXIS2_PLACEMENT_3D ( 'NONE', #6030, #5194, #5247 ) ;
#9051=VECTOR ( 'NONE', #3123, 1000.000000000000000 ) ;
#9064=APPLICATION_CONTEXT ( 'automotive_design' ) ;
#9065=SHAPE_REPRESENTATION_RELATIONSHIP ( 'NONE' , 'NONE' ,  #6499, #8040 ) ;
#9067=ORIENTED_EDGE ( 'NONE', *, *, #8054, .F. ) ;
#9070=DIRECTION ( 'NONE',  ( 1.156482317317871478E-16, -1.000000000000000000, -0.000000000000000000 ) ) ;
#9079=CARTESIAN_POINT ( 'NONE',  ( 27.00000000000001066, 35.00000000000001421, 5.999999999999999112 ) ) ;
#9090=ORIENTED_EDGE ( 'NONE', *, *, #2457, .T. ) ;
#9094=CARTESIAN_POINT ( 'NONE',  ( -29.99999999999998934, -13.00000000000000533, -1.249999999999993339 ) ) ;
#9102=VERTEX_POINT ( 'NONE', #8632 ) ;
#9123=LINE ( 'NONE', #1863, #8992 ) ;
#9137=ORIENTED_EDGE ( 'NONE', *, *, #9940, .F. ) ;
#9147=AXIS2_PLACEMENT_3D ( 'NONE', #10311, #1243, #4467 ) ;
#9148=ADVANCED_FACE ( 'NONE', ( #523 ), #9440, .F. ) ;
#9151=ORIENTED_EDGE ( 'NONE', *, *, #7899, .T. ) ;
#9188=FACE_OUTER_BOUND ( 'NONE', #8351, .T. ) ;
#9194=CARTESIAN_POINT ( 'NONE',  ( 30.00000000000001066, 35.00000000000001421, -6.000000000000000000 ) ) ;
#9197=VERTEX_POINT ( 'NONE', #7308 ) ;
#9208=DIRECTION ( 'NONE',  ( 1.000000000000000000, 0.000000000000000000, 0.000000000000000000 ) ) ;
#9221=DIRECTION ( 'NONE',  ( -1.000000000000000000, -1.156482317317871478E-16, -5.694029147589358720E-15 ) ) ;
#9223=DIRECTION ( 'NONE',  ( 1.000000000000000000, -0.000000000000000000, -0.000000000000000000 ) ) ;
#9252=AXIS2_PLACEMENT_3D ( 'NONE', #585, #4708, #696 ) ;
#9269=ORIENTED_EDGE ( 'NONE', *, *, #1377, .T. ) ;
#9308=CARTESIAN_POINT ( 'NONE',  ( -29.99999999999998934, -35.00000000000000000, 9.000000000000000000 ) ) ;
#9310=CARTESIAN_POINT ( 'NONE',  ( 7.054542135639013677E-15, -28.99999999999999289, 0.000000000000000000 ) ) ;
#9311=ORIENTED_EDGE ( 'NONE', *, *, #6815, .T. ) ;
#9323=ORIENTED_EDGE ( 'NONE', *, *, #10242, .F. ) ;
#9331=EDGE_CURVE ( 'NONE', #3641, #5372, #1590, .T. ) ;
#9340=CARTESIAN_POINT ( 'NONE',  ( -29.99999999999998934, -13.00000000000000533, 0.000000000000000000 ) ) ;
#9350=ORIENTED_EDGE ( 'NONE', *, *, #3234, .T. ) ;
#9372=CYLINDRICAL_SURFACE ( 'NONE', #668, 2.000000000000001776 ) ;
#9402=VECTOR ( 'NONE', #1803, 1000.000000000000000 ) ;
#9412=CARTESIAN_POINT ( 'NONE',  ( -1.387778780781445991E-14, 15.00000000000000355, 0.000000000000000000 ) ) ;
#9416=ADVANCED_FACE ( 'NONE', ( #6934 ), #278, .F. ) ;
#9420=VERTEX_POINT ( 'NONE', #7693 ) ;
#9421=AXIS2_PLACEMENT_3D ( 'NONE', #7562, #7667, #6054 ) ;
#9439=DIRECTION ( 'NONE',  ( 1.000000000000000000, 2.312964634635742957E-16, -0.000000000000000000 ) ) ;
#9440=CYLINDRICAL_SURFACE ( 'NONE', #730, 2.000000000000001776 ) ;
#9448=DIRECTION ( 'NONE',  ( -1.000000000000000000, -1.156482317317871478E-16, 5.204170427930421283E-15 ) ) ;
#9449=DIRECTION ( 'NONE',  ( 0.000000000000000000, 0.000000000000000000, -1.000000000000000000 ) ) ;
#9461=DIRECTION ( 'NONE',  ( -1.000000000000000000, -4.625929269271485914E-16, 0.000000000000000000 ) ) ;
#9469=EDGE_LOOP ( 'NONE', ( #9968, #459, #7159, #426 ) ) ;
#9472=FACE_OUTER_BOUND ( 'NONE', #8106, .T. ) ;
#9484=AXIS2_PLACEMENT_3D ( 'NONE', #5766, #8172, #7417 ) ;
#9488=CARTESIAN_POINT ( 'NONE',  ( 27.00000000000001066, -34.99999999999999289, -6.000000000000000000 ) ) ;
#9492=DIRECTION ( 'NONE',  ( -0.000000000000000000, -0.000000000000000000, 1.000000000000000000 ) ) ;
#9495=AXIS2_PLACEMENT_3D ( 'NONE', #9862, #8162, #1793 ) ;
#9501=CIRCLE ( 'NONE', #3905, 2.500000000000000000 ) ;
#9512=FACE_BOUND ( 'NONE', #5706, .T. ) ;
#9516=EDGE_CURVE ( 'NONE', #9197, #409, #2280, .T. ) ;
#9517=CARTESIAN_POINT ( 'NONE',  ( 1.999999999999973577, 35.00000000000000000, -6.000000000000009770 ) ) ;
#9519=LINE ( 'NONE', #8029, #953 ) ;
#9523=EDGE_CURVE ( 'NONE', #9197, #2891, #3020, .T. ) ;
#9528=EDGE_CURVE ( 'NONE', #8329, #2528, #5801, .T. ) ;
#9529=VERTEX_POINT ( 'NONE', #5554 ) ;
#9535=FACE_OUTER_BOUND ( 'NONE', #3696, .T. ) ;
#9543=VERTEX_POINT ( 'NONE', #8744 ) ;
#9558=( GEOMETRIC_REPRESENTATION_CONTEXT ( 3 ) GLOBAL_UNCERTAINTY_ASSIGNED_CONTEXT ( ( #465 ) ) GLOBAL_UNIT_ASSIGNED_CONTEXT ( ( #9812, #1596, #6560 ) ) REPRESENTATION_CONTEXT ( 'NONE', 'WORKASPACE' ) );
#9585=VERTEX_POINT ( 'NONE', #6239 ) ;
#9604=CARTESIAN_POINT ( 'NONE',  ( -15.00000000000000000, 19.99999999999999645, -9.000000000000000000 ) ) ;
#9623=LINE ( 'NONE', #6416, #1963 ) ;
#9625=DIRECTION ( 'NONE',  ( 1.000000000000000000, 1.156482317317871478E-16, -5.204170427930421283E-15 ) ) ;
#9630=DIRECTION ( 'NONE',  ( -0.000000000000000000, -0.000000000000000000, 1.000000000000000000 ) ) ;
#9634=ORIENTED_EDGE ( 'NONE', *, *, #8689, .T. ) ;
#9644=ORIENTED_EDGE ( 'NONE', *, *, #9331, .T. ) ;
#9652=CARTESIAN_POINT ( 'NONE',  ( -2.000000000000024425, 15.00000000000000355, -5.999999999999988454 ) ) ;
#9654=VERTEX_POINT ( 'NONE', #8360 ) ;
#9656=EDGE_CURVE ( 'NONE', #9420, #6021, #3425, .T. ) ;
#9672=AXIS2_PLACEMENT_3D ( 'NONE', #3965, #7194, #4643 ) ;
#9687=PLANE ( 'NONE',  #183 ) ;
#9694=EDGE_CURVE ( 'NONE', #6538, #3281, #2257, .T. ) ;
#9703=EDGE_CURVE ( 'NONE', #9040, #8624, #5746, .T. ) ;
#9730=CARTESIAN_POINT ( 'NONE',  ( 15.00000000000000000, 19.99999999999999645, -9.000000000000000000 ) ) ;
#9735=CIRCLE ( 'NONE', #1085, 1.249999999999987121 ) ;
#9764=CIRCLE ( 'NONE', #10100, 2.000000000000000000 ) ;
#9781=FACE_OUTER_BOUND ( 'NONE', #1505, .T. ) ;
#9803=CARTESIAN_POINT ( 'NONE',  ( -29.99999999999998934, -35.00000000000000000, 9.000000000000000000 ) ) ;
#9804=EDGE_CURVE ( 'NONE', #3277, #9040, #2441, .T. ) ;
#9805=LINE ( 'NONE', #5021, #10344 ) ;
#9806=VERTEX_POINT ( 'NONE', #6638 ) ;
#9812=( LENGTH_UNIT ( ) NAMED_UNIT ( * ) SI_UNIT ( .MILLI., .METRE. ) );
#9817=DIRECTION ( 'NONE',  ( -0.000000000000000000, -0.000000000000000000, 1.000000000000000000 ) ) ;
#9821=VERTEX_POINT ( 'NONE', #8194 ) ;
#9835=CARTESIAN_POINT ( 'NONE',  ( 30.00000000000001066, 0.000000000000000000, 0.000000000000000000 ) ) ;
#9838=CARTESIAN_POINT ( 'NONE',  ( -26.99999999999998934, -35.00000000000000000, 5.999999999999999112 ) ) ;
#9846=ADVANCED_FACE ( 'NONE', ( #1877, #3415, #8984 ), #82, .F. ) ;
#9850=VERTEX_POINT ( 'NONE', #7496 ) ;
#9856=AXIS2_PLACEMENT_3D ( 'NONE', #8517, #1251, #6965 ) ;
#9860=EDGE_LOOP ( 'NONE', ( #5611, #9311, #4430, #7789 ) ) ;
#9861=CARTESIAN_POINT ( 'NONE',  ( 15.00000000000000000, 19.99999999999999645, 9.000000000000000000 ) ) ;
#9862=CARTESIAN_POINT ( 'NONE',  ( -1.387778780781445991E-14, 15.00000000000000355, 0.000000000000000000 ) ) ;
#9863=ORIENTED_EDGE ( 'NONE', *, *, #2948, .T. ) ;
#9868=EDGE_CURVE ( 'NONE', #3947, #317, #4153, .T. ) ;
#9874=DIRECTION ( 'NONE',  ( 0.000000000000000000, 0.000000000000000000, -1.000000000000000000 ) ) ;
#9878=CARTESIAN_POINT ( 'NONE',  ( 17.00000000000000000, 19.99999999999999645, 9.000000000000000000 ) ) ;
#9892=AXIS2_PLACEMENT_3D ( 'NONE', #1772, #4949, #5729 ) ;
#9896=CARTESIAN_POINT ( 'NONE',  ( 30.00000000000001066, 35.00000000000001421, 9.000000000000000000 ) ) ;
#9902=VERTEX_POINT ( 'NONE', #6895 ) ;
#9904=DIRECTION ( 'NONE',  ( -0.000000000000000000, -0.000000000000000000, 1.000000000000000000 ) ) ;
#9933=CARTESIAN_POINT ( 'NONE',  ( 12.99999999999999645, 19.99999999999999645, -9.000000000000000000 ) ) ;
#9939=PLANE ( 'NONE',  #8402 ) ;
#9940=EDGE_CURVE ( 'NONE', #9979, #317, #3031, .T. ) ;
#9943=CYLINDRICAL_SURFACE ( 'NONE', #2722, 2.000000000000000000 ) ;
#9962=CARTESIAN_POINT ( 'NONE',  ( -17.00000000000000000, 19.99999999999999645, -5.999999999999999112 ) ) ;
#9968=ORIENTED_EDGE ( 'NONE', *, *, #10126, .F. ) ;
#9979=VERTEX_POINT ( 'NONE', #3822 ) ;
#9981=DIRECTION ( 'NONE',  ( -0.000000000000000000, -0.000000000000000000, 1.000000000000000000 ) ) ;
#9983=FACE_OUTER_BOUND ( 'NONE', #4878, .T. ) ;
#9994=DIRECTION ( 'NONE',  ( -1.000000000000000000, 0.000000000000000000, 0.000000000000000000 ) ) ;
#10025=ADVANCED_FACE ( 'NONE', ( #7158, #9512, #10416 ), #1389, .F. ) ;
#10029=VECTOR ( 'NONE', #6485, 1000.000000000000000 ) ;
#10040=DIRECTION ( 'NONE',  ( -2.312964634635742957E-16, 1.000000000000000000, 0.000000000000000000 ) ) ;
#10052=DIRECTION ( 'NONE',  ( 1.000000000000000000, 0.000000000000000000, 0.000000000000000000 ) ) ;
#10066=EDGE_CURVE ( 'NONE', #8624, #4919, #1242, .T. ) ;
#10075=DIRECTION ( 'NONE',  ( -1.000000000000000000, -0.000000000000000000, -0.000000000000000000 ) ) ;
#10077=PLANE ( 'NONE',  #7272 ) ;
#10084=ORIENTED_EDGE ( 'NONE', *, *, #1069, .T. ) ;
#10086=CARTESIAN_POINT ( 'NONE',  ( 7.054542135639013677E-15, -28.99999999999999289, 0.000000000000000000 ) ) ;
#10091=VECTOR ( 'NONE', #4488, 1000.000000000000000 ) ;
#10100=AXIS2_PLACEMENT_3D ( 'NONE', #6796, #7654, #10052 ) ;
#10105=ORIENTED_EDGE ( 'NONE', *, *, #2457, .F. ) ;
#10126=EDGE_CURVE ( 'NONE', #3277, #4919, #1656, .T. ) ;
#10136=ORIENTED_EDGE ( 'NONE', *, *, #2803, .F. ) ;
#10144=CARTESIAN_POINT ( 'NONE',  ( -29.99999999999998934, -13.00000000000000533, 0.000000000000000000 ) ) ;
#10150=ORIENTED_EDGE ( 'NONE', *, *, #5357, .T. ) ;
#10166=FACE_OUTER_BOUND ( 'NONE', #7706, .T. ) ;
#10167=ORIENTED_EDGE ( 'NONE', *, *, #6493, .F. ) ;
#10188=VERTEX_POINT ( 'NONE', #9079 ) ;
#10201=EDGE_CURVE ( 'NONE', #6622, #6819, #576, .T. ) ;
#10210=ORIENTED_EDGE ( 'NONE', *, *, #6737, .F. ) ;
#10216=ORIENTED_EDGE ( 'NONE', *, *, #2362, .T. ) ;
#10217=ORIENTED_EDGE ( 'NONE', *, *, #7626, .T. ) ;
#10220=CARTESIAN_POINT ( 'NONE',  ( 15.00000000000000000, 19.99999999999999645, 6.000000000000000000 ) ) ;
#10227=ORIENTED_EDGE ( 'NONE', *, *, #4084, .T. ) ;
#10231=CARTESIAN_POINT ( 'NONE',  ( -2.000000000000012879, 15.00000000000000355, 3.999999999999986233 ) ) ;
#10242=EDGE_CURVE ( 'NONE', #2444, #7878, #9735, .T. ) ;
#10244=FACE_BOUND ( 'NONE', #2404, .T. ) ;
#10245=DIRECTION ( 'NONE',  ( -1.000000000000000000, -1.156482317317871478E-16, 5.204170427930421283E-15 ) ) ;
#10246=CARTESIAN_POINT ( 'NONE',  ( 17.00000000000000000, 19.99999999999999645, -9.000000000000000000 ) ) ;
#10256=EDGE_CURVE ( 'NONE', #7878, #2444, #5309, .T. ) ;
#10264=AXIS2_PLACEMENT_3D ( 'NONE', #2766, #6787, #5980 ) ;
#10296=ADVANCED_FACE ( 'NONE', ( #9983, #1166, #1222 ), #8591, .T. ) ;
#10307=PLANE ( 'NONE',  #1285 ) ;
#10310=CARTESIAN_POINT ( 'NONE',  ( -2.000000000000024425, 15.00000000000000355, -5.999999999999988454 ) ) ;
#10311=CARTESIAN_POINT ( 'NONE',  ( -15.00000000000000000, 19.99999999999999645, -9.000000000000000000 ) ) ;
#10321=VECTOR ( 'NONE', #7387, 1000.000000000000000 ) ;
#10344=VECTOR ( 'NONE', #4218, 1000.000000000000000 ) ;
#10347=CARTESIAN_POINT ( 'NONE',  ( 30.00000000000001066, -34.99999999999999289, 9.000000000000000000 ) ) ;
#10370=CARTESIAN_POINT ( 'NONE',  ( 12.99999999999999645, 19.99999999999999645, -9.000000000000000000 ) ) ;
#10380=EDGE_CURVE ( 'NONE', #5808, #4718, #1936, .T. ) ;
#10385=CYLINDRICAL_SURFACE ( 'NONE', #1855, 1.999999999999997780 ) ;
#10396=DIRECTION ( 'NONE',  ( 0.000000000000000000, 1.000000000000000000, 0.000000000000000000 ) ) ;
#10398=LINE ( 'NONE', #3117, #3540 ) ;
#10408=CARTESIAN_POINT ( 'NONE',  ( 1.999999999999986233, 15.00000000000000355, -4.000000000000009770 ) ) ;
#10416=FACE_OUTER_BOUND ( 'NONE', #3912, .T. ) ;
#10417=EDGE_LOOP ( 'NONE', ( #1306, #8023 ) ) ;
#10436=VECTOR ( 'NONE', #2892, 1000.000000000000000 ) ;
#10442=ORIENTED_EDGE ( 'NONE', *, *, #8813, .T. ) ;
#10447=ORIENTED_EDGE ( 'NONE', *, *, #8134, .T. ) ;
#10448=CIRCLE ( 'NONE', #7722, 2.500000000000000000 ) ;
ENDSEC;
END-ISO-10303-21;
